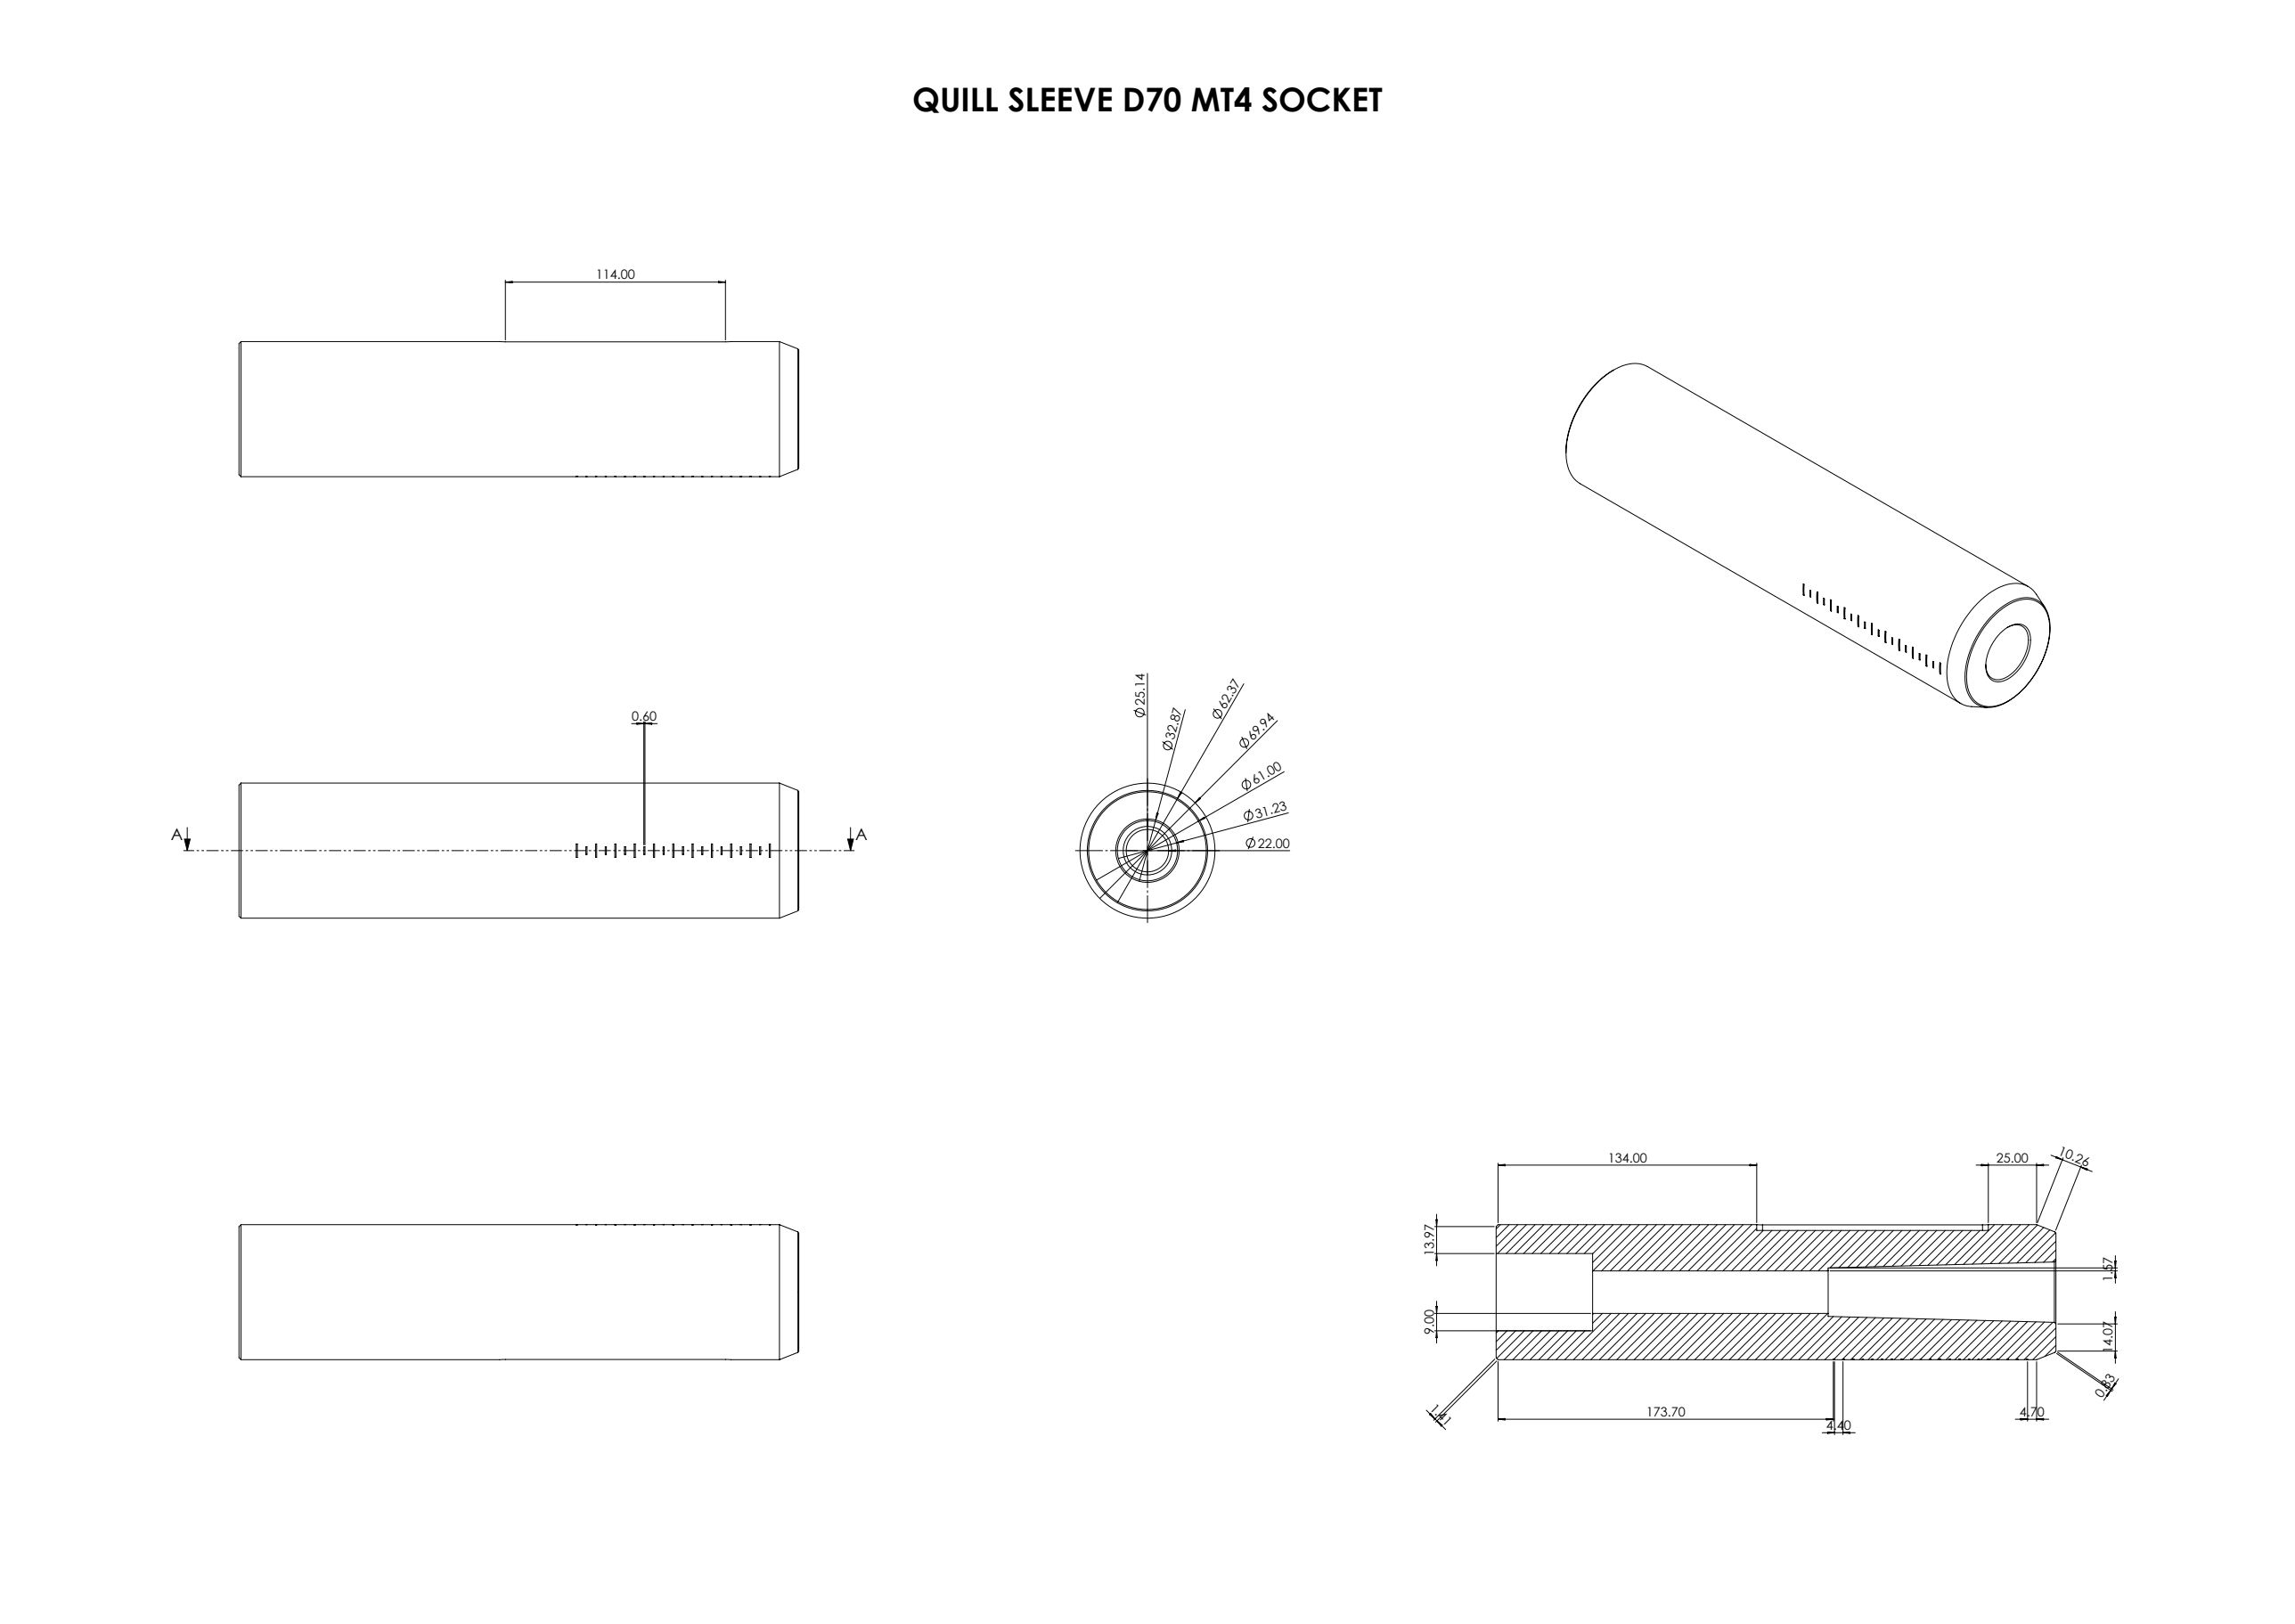
ISO-10303-21;
HEADER;
/* Generated by software containing ST-Developer
 * from STEP Tools, Inc. (www.steptools.com) 
 */

FILE_DESCRIPTION(
/* description */ (''),
/* implementation_level */ '2;1');

FILE_NAME(
/* name */ '03_Quill_Sleeve_D70_MT4_Socket.step',
/* time_stamp */ '2026-10-26T03:50:32-07:00',
/* author */ (''),
/* organization */ (''),
/* preprocessor_version */ 'ST-DEVELOPER v20.2',
/* originating_system */ 'Autodesk Translation Framework v15.15.0.0',
/* authorisation */ '');

FILE_SCHEMA (('AUTOMOTIVE_DESIGN { 1 0 10303 214 3 1 1 }'));
ENDSEC;

DATA;
#10=MECHANICAL_DESIGN_GEOMETRIC_PRESENTATION_REPRESENTATION('',(#1041),#76660);
#237=B_SPLINE_CURVE_WITH_KNOTS('',3,(#39988,#39989,#39990,#39991,#39992,
#39993,#39994,#39995,#39996,#39997,#39998,#39999,#40000,#40001,#40002,#40003,
#40004,#40005),.UNSPECIFIED.,.F.,.F.,(4,2,2,2,2,2,2,2,4),(0.,0.113065755992561,
0.226131511985123,0.3391970600484,0.452262608111676,0.565328156174953,0.67839370423823,
0.791459460230791,0.904525216223353),.UNSPECIFIED.);
#238=B_SPLINE_CURVE_WITH_KNOTS('',3,(#40016,#40017,#40018,#40019,#40020,
#40021,#40022,#40023,#40024,#40025,#40026,#40027,#40028,#40029,#40030,#40031,
#40032,#40033),.UNSPECIFIED.,.F.,.F.,(4,2,2,2,2,2,2,2,4),(-0.904525216223347,
-0.791459460230787,-0.678393704238228,-0.565328156174951,-0.452262608111673,
-0.339197060048396,-0.226131511985119,-0.11306575599256,0.),
 .UNSPECIFIED.);
#1001=SHAPE_REPRESENTATION_RELATIONSHIP('SRR','None',#76738,#1021);
#1021=ADVANCED_BREP_SHAPE_REPRESENTATION('',(#1061),#76642);
#1041=STYLED_ITEM('',(#76920),#1061);
#1061=MANIFOLD_SOLID_BREP('Quill',#26666);
#1155=CYLINDRICAL_SURFACE('',#27552,0.3);
#1156=CYLINDRICAL_SURFACE('',#27555,0.3);
#1157=CYLINDRICAL_SURFACE('',#27558,2.);
#1158=CYLINDRICAL_SURFACE('',#27565,3.497);
#1159=CYLINDRICAL_SURFACE('',#27572,1.1);
#1580=FACE_BOUND('',#4415,.T.);
#1581=FACE_BOUND('',#4528,.T.);
#1582=FACE_BOUND('',#4531,.T.);
#1583=FACE_BOUND('',#4532,.T.);
#1584=FACE_BOUND('',#4533,.T.);
#1585=FACE_BOUND('',#4534,.T.);
#1586=FACE_BOUND('',#4535,.T.);
#1587=FACE_BOUND('',#4536,.T.);
#1588=FACE_BOUND('',#4537,.T.);
#1589=FACE_BOUND('',#4538,.T.);
#1590=FACE_BOUND('',#4539,.T.);
#1591=FACE_BOUND('',#4540,.T.);
#1592=FACE_BOUND('',#4541,.T.);
#1593=FACE_BOUND('',#4542,.T.);
#1594=FACE_BOUND('',#4543,.T.);
#1595=FACE_BOUND('',#4544,.T.);
#1596=FACE_BOUND('',#4545,.T.);
#1597=FACE_BOUND('',#4546,.T.);
#1598=FACE_BOUND('',#4547,.T.);
#1599=FACE_BOUND('',#4548,.T.);
#1600=FACE_BOUND('',#4549,.T.);
#1601=FACE_BOUND('',#4550,.T.);
#1602=FACE_BOUND('',#4551,.T.);
#1603=FACE_BOUND('',#4552,.T.);
#1604=FACE_BOUND('',#4556,.T.);
#1605=FACE_BOUND('',#4559,.T.);
#1804=PLANE('',#27402);
#1805=PLANE('',#27404);
#1806=PLANE('',#27405);
#1807=PLANE('',#27407);
#1808=PLANE('',#27408);
#1809=PLANE('',#27410);
#1810=PLANE('',#27411);
#1811=PLANE('',#27412);
#1812=PLANE('',#27414);
#1813=PLANE('',#27415);
#1814=PLANE('',#27417);
#1815=PLANE('',#27418);
#1816=PLANE('',#27419);
#1817=PLANE('',#27421);
#1818=PLANE('',#27422);
#1819=PLANE('',#27424);
#1820=PLANE('',#27425);
#1821=PLANE('',#27426);
#1822=PLANE('',#27428);
#1823=PLANE('',#27429);
#1824=PLANE('',#27431);
#1825=PLANE('',#27432);
#1826=PLANE('',#27433);
#1827=PLANE('',#27435);
#1828=PLANE('',#27436);
#1829=PLANE('',#27438);
#1830=PLANE('',#27439);
#1831=PLANE('',#27440);
#1832=PLANE('',#27442);
#1833=PLANE('',#27443);
#1834=PLANE('',#27445);
#1835=PLANE('',#27446);
#1836=PLANE('',#27447);
#1837=PLANE('',#27449);
#1838=PLANE('',#27450);
#1839=PLANE('',#27452);
#1840=PLANE('',#27453);
#1841=PLANE('',#27454);
#1842=PLANE('',#27456);
#1843=PLANE('',#27457);
#1844=PLANE('',#27459);
#1845=PLANE('',#27460);
#1846=PLANE('',#27461);
#1847=PLANE('',#27463);
#1848=PLANE('',#27464);
#1849=PLANE('',#27466);
#1850=PLANE('',#27467);
#1851=PLANE('',#27468);
#1852=PLANE('',#27470);
#1853=PLANE('',#27471);
#1854=PLANE('',#27473);
#1855=PLANE('',#27474);
#1856=PLANE('',#27475);
#1857=PLANE('',#27477);
#1858=PLANE('',#27478);
#1859=PLANE('',#27480);
#1860=PLANE('',#27481);
#1861=PLANE('',#27482);
#1862=PLANE('',#27484);
#1863=PLANE('',#27485);
#1864=PLANE('',#27487);
#1865=PLANE('',#27488);
#1866=PLANE('',#27489);
#1867=PLANE('',#27491);
#1868=PLANE('',#27492);
#1869=PLANE('',#27494);
#1870=PLANE('',#27495);
#1871=PLANE('',#27496);
#1872=PLANE('',#27498);
#1873=PLANE('',#27499);
#1874=PLANE('',#27501);
#1875=PLANE('',#27502);
#1876=PLANE('',#27503);
#1877=PLANE('',#27505);
#1878=PLANE('',#27506);
#1879=PLANE('',#27508);
#1880=PLANE('',#27509);
#1881=PLANE('',#27510);
#1882=PLANE('',#27512);
#1883=PLANE('',#27513);
#1884=PLANE('',#27515);
#1885=PLANE('',#27516);
#1886=PLANE('',#27517);
#1887=PLANE('',#27519);
#1888=PLANE('',#27520);
#1889=PLANE('',#27522);
#1890=PLANE('',#27523);
#1891=PLANE('',#27524);
#1892=PLANE('',#27526);
#1893=PLANE('',#27527);
#1894=PLANE('',#27529);
#1895=PLANE('',#27530);
#1896=PLANE('',#27531);
#1897=PLANE('',#27533);
#1898=PLANE('',#27534);
#1899=PLANE('',#27536);
#1900=PLANE('',#27537);
#1901=PLANE('',#27538);
#1902=PLANE('',#27540);
#1903=PLANE('',#27541);
#1904=PLANE('',#27543);
#1905=PLANE('',#27544);
#1906=PLANE('',#27545);
#1907=PLANE('',#27547);
#1908=PLANE('',#27548);
#1909=PLANE('',#27550);
#1910=PLANE('',#27551);
#1911=PLANE('',#27554);
#1912=PLANE('',#27557);
#1913=PLANE('',#27561);
#1914=PLANE('',#27570);
#1915=PLANE('',#27574);
#2833=FACE_OUTER_BOUND('',#4412,.T.);
#2834=FACE_OUTER_BOUND('',#4413,.T.);
#2835=FACE_OUTER_BOUND('',#4414,.T.);
#2836=FACE_OUTER_BOUND('',#4416,.T.);
#2837=FACE_OUTER_BOUND('',#4417,.T.);
#2838=FACE_OUTER_BOUND('',#4418,.T.);
#2839=FACE_OUTER_BOUND('',#4419,.T.);
#2840=FACE_OUTER_BOUND('',#4420,.T.);
#2841=FACE_OUTER_BOUND('',#4421,.T.);
#2842=FACE_OUTER_BOUND('',#4422,.T.);
#2843=FACE_OUTER_BOUND('',#4423,.T.);
#2844=FACE_OUTER_BOUND('',#4424,.T.);
#2845=FACE_OUTER_BOUND('',#4425,.T.);
#2846=FACE_OUTER_BOUND('',#4426,.T.);
#2847=FACE_OUTER_BOUND('',#4427,.T.);
#2848=FACE_OUTER_BOUND('',#4428,.T.);
#2849=FACE_OUTER_BOUND('',#4429,.T.);
#2850=FACE_OUTER_BOUND('',#4430,.T.);
#2851=FACE_OUTER_BOUND('',#4431,.T.);
#2852=FACE_OUTER_BOUND('',#4432,.T.);
#2853=FACE_OUTER_BOUND('',#4433,.T.);
#2854=FACE_OUTER_BOUND('',#4434,.T.);
#2855=FACE_OUTER_BOUND('',#4435,.T.);
#2856=FACE_OUTER_BOUND('',#4436,.T.);
#2857=FACE_OUTER_BOUND('',#4437,.T.);
#2858=FACE_OUTER_BOUND('',#4438,.T.);
#2859=FACE_OUTER_BOUND('',#4439,.T.);
#2860=FACE_OUTER_BOUND('',#4440,.T.);
#2861=FACE_OUTER_BOUND('',#4441,.T.);
#2862=FACE_OUTER_BOUND('',#4442,.T.);
#2863=FACE_OUTER_BOUND('',#4443,.T.);
#2864=FACE_OUTER_BOUND('',#4444,.T.);
#2865=FACE_OUTER_BOUND('',#4445,.T.);
#2866=FACE_OUTER_BOUND('',#4446,.T.);
#2867=FACE_OUTER_BOUND('',#4447,.T.);
#2868=FACE_OUTER_BOUND('',#4448,.T.);
#2869=FACE_OUTER_BOUND('',#4449,.T.);
#2870=FACE_OUTER_BOUND('',#4450,.T.);
#2871=FACE_OUTER_BOUND('',#4451,.T.);
#2872=FACE_OUTER_BOUND('',#4452,.T.);
#2873=FACE_OUTER_BOUND('',#4453,.T.);
#2874=FACE_OUTER_BOUND('',#4454,.T.);
#2875=FACE_OUTER_BOUND('',#4455,.T.);
#2876=FACE_OUTER_BOUND('',#4456,.T.);
#2877=FACE_OUTER_BOUND('',#4457,.T.);
#2878=FACE_OUTER_BOUND('',#4458,.T.);
#2879=FACE_OUTER_BOUND('',#4459,.T.);
#2880=FACE_OUTER_BOUND('',#4460,.T.);
#2881=FACE_OUTER_BOUND('',#4461,.T.);
#2882=FACE_OUTER_BOUND('',#4462,.T.);
#2883=FACE_OUTER_BOUND('',#4463,.T.);
#2884=FACE_OUTER_BOUND('',#4464,.T.);
#2885=FACE_OUTER_BOUND('',#4465,.T.);
#2886=FACE_OUTER_BOUND('',#4466,.T.);
#2887=FACE_OUTER_BOUND('',#4467,.T.);
#2888=FACE_OUTER_BOUND('',#4468,.T.);
#2889=FACE_OUTER_BOUND('',#4469,.T.);
#2890=FACE_OUTER_BOUND('',#4470,.T.);
#2891=FACE_OUTER_BOUND('',#4471,.T.);
#2892=FACE_OUTER_BOUND('',#4472,.T.);
#2893=FACE_OUTER_BOUND('',#4473,.T.);
#2894=FACE_OUTER_BOUND('',#4474,.T.);
#2895=FACE_OUTER_BOUND('',#4475,.T.);
#2896=FACE_OUTER_BOUND('',#4476,.T.);
#2897=FACE_OUTER_BOUND('',#4477,.T.);
#2898=FACE_OUTER_BOUND('',#4478,.T.);
#2899=FACE_OUTER_BOUND('',#4479,.T.);
#2900=FACE_OUTER_BOUND('',#4480,.T.);
#2901=FACE_OUTER_BOUND('',#4481,.T.);
#2902=FACE_OUTER_BOUND('',#4482,.T.);
#2903=FACE_OUTER_BOUND('',#4483,.T.);
#2904=FACE_OUTER_BOUND('',#4484,.T.);
#2905=FACE_OUTER_BOUND('',#4485,.T.);
#2906=FACE_OUTER_BOUND('',#4486,.T.);
#2907=FACE_OUTER_BOUND('',#4487,.T.);
#2908=FACE_OUTER_BOUND('',#4488,.T.);
#2909=FACE_OUTER_BOUND('',#4489,.T.);
#2910=FACE_OUTER_BOUND('',#4490,.T.);
#2911=FACE_OUTER_BOUND('',#4491,.T.);
#2912=FACE_OUTER_BOUND('',#4492,.T.);
#2913=FACE_OUTER_BOUND('',#4493,.T.);
#2914=FACE_OUTER_BOUND('',#4494,.T.);
#2915=FACE_OUTER_BOUND('',#4495,.T.);
#2916=FACE_OUTER_BOUND('',#4496,.T.);
#2917=FACE_OUTER_BOUND('',#4497,.T.);
#2918=FACE_OUTER_BOUND('',#4498,.T.);
#2919=FACE_OUTER_BOUND('',#4499,.T.);
#2920=FACE_OUTER_BOUND('',#4500,.T.);
#2921=FACE_OUTER_BOUND('',#4501,.T.);
#2922=FACE_OUTER_BOUND('',#4502,.T.);
#2923=FACE_OUTER_BOUND('',#4503,.T.);
#2924=FACE_OUTER_BOUND('',#4504,.T.);
#2925=FACE_OUTER_BOUND('',#4505,.T.);
#2926=FACE_OUTER_BOUND('',#4506,.T.);
#2927=FACE_OUTER_BOUND('',#4507,.T.);
#2928=FACE_OUTER_BOUND('',#4508,.T.);
#2929=FACE_OUTER_BOUND('',#4509,.T.);
#2930=FACE_OUTER_BOUND('',#4510,.T.);
#2931=FACE_OUTER_BOUND('',#4511,.T.);
#2932=FACE_OUTER_BOUND('',#4512,.T.);
#2933=FACE_OUTER_BOUND('',#4513,.T.);
#2934=FACE_OUTER_BOUND('',#4514,.T.);
#2935=FACE_OUTER_BOUND('',#4515,.T.);
#2936=FACE_OUTER_BOUND('',#4516,.T.);
#2937=FACE_OUTER_BOUND('',#4517,.T.);
#2938=FACE_OUTER_BOUND('',#4518,.T.);
#2939=FACE_OUTER_BOUND('',#4519,.T.);
#2940=FACE_OUTER_BOUND('',#4520,.T.);
#2941=FACE_OUTER_BOUND('',#4521,.T.);
#2942=FACE_OUTER_BOUND('',#4522,.T.);
#2943=FACE_OUTER_BOUND('',#4523,.T.);
#2944=FACE_OUTER_BOUND('',#4524,.T.);
#2945=FACE_OUTER_BOUND('',#4525,.T.);
#2946=FACE_OUTER_BOUND('',#4526,.T.);
#2947=FACE_OUTER_BOUND('',#4527,.T.);
#2948=FACE_OUTER_BOUND('',#4529,.T.);
#2949=FACE_OUTER_BOUND('',#4530,.T.);
#2950=FACE_OUTER_BOUND('',#4553,.T.);
#2951=FACE_OUTER_BOUND('',#4554,.T.);
#2952=FACE_OUTER_BOUND('',#4555,.T.);
#2953=FACE_OUTER_BOUND('',#4557,.T.);
#2954=FACE_OUTER_BOUND('',#4558,.T.);
#4412=EDGE_LOOP('',(#18651,#18652,#18653,#18654,#18655));
#4413=EDGE_LOOP('',(#18656,#18657,#18658,#18659,#18660));
#4414=EDGE_LOOP('',(#18661));
#4415=EDGE_LOOP('',(#18662));
#4416=EDGE_LOOP('',(#18663,#18664,#18665,#18666));
#4417=EDGE_LOOP('',(#18667,#18668,#18669,#18670));
#4418=EDGE_LOOP('',(#18671,#18672,#18673,#18674));
#4419=EDGE_LOOP('',(#18675,#18676,#18677,#18678));
#4420=EDGE_LOOP('',(#18679,#18680,#18681,#18682));
#4421=EDGE_LOOP('',(#18683,#18684,#18685,#18686));
#4422=EDGE_LOOP('',(#18687,#18688,#18689,#18690));
#4423=EDGE_LOOP('',(#18691,#18692,#18693,#18694));
#4424=EDGE_LOOP('',(#18695,#18696,#18697,#18698));
#4425=EDGE_LOOP('',(#18699,#18700,#18701,#18702));
#4426=EDGE_LOOP('',(#18703,#18704,#18705,#18706));
#4427=EDGE_LOOP('',(#18707,#18708,#18709,#18710));
#4428=EDGE_LOOP('',(#18711,#18712,#18713,#18714));
#4429=EDGE_LOOP('',(#18715,#18716,#18717,#18718));
#4430=EDGE_LOOP('',(#18719,#18720,#18721,#18722));
#4431=EDGE_LOOP('',(#18723,#18724,#18725,#18726));
#4432=EDGE_LOOP('',(#18727,#18728,#18729,#18730));
#4433=EDGE_LOOP('',(#18731,#18732,#18733,#18734));
#4434=EDGE_LOOP('',(#18735,#18736,#18737,#18738));
#4435=EDGE_LOOP('',(#18739,#18740,#18741,#18742));
#4436=EDGE_LOOP('',(#18743,#18744,#18745,#18746));
#4437=EDGE_LOOP('',(#18747,#18748,#18749,#18750));
#4438=EDGE_LOOP('',(#18751,#18752,#18753,#18754));
#4439=EDGE_LOOP('',(#18755,#18756,#18757,#18758));
#4440=EDGE_LOOP('',(#18759,#18760,#18761,#18762));
#4441=EDGE_LOOP('',(#18763,#18764,#18765,#18766));
#4442=EDGE_LOOP('',(#18767,#18768,#18769,#18770));
#4443=EDGE_LOOP('',(#18771,#18772,#18773,#18774));
#4444=EDGE_LOOP('',(#18775,#18776,#18777,#18778));
#4445=EDGE_LOOP('',(#18779,#18780,#18781,#18782));
#4446=EDGE_LOOP('',(#18783,#18784,#18785,#18786));
#4447=EDGE_LOOP('',(#18787,#18788,#18789,#18790));
#4448=EDGE_LOOP('',(#18791,#18792,#18793,#18794));
#4449=EDGE_LOOP('',(#18795,#18796,#18797,#18798));
#4450=EDGE_LOOP('',(#18799,#18800,#18801,#18802));
#4451=EDGE_LOOP('',(#18803,#18804,#18805,#18806));
#4452=EDGE_LOOP('',(#18807,#18808,#18809,#18810));
#4453=EDGE_LOOP('',(#18811,#18812,#18813,#18814));
#4454=EDGE_LOOP('',(#18815,#18816,#18817,#18818));
#4455=EDGE_LOOP('',(#18819,#18820,#18821,#18822));
#4456=EDGE_LOOP('',(#18823,#18824,#18825,#18826));
#4457=EDGE_LOOP('',(#18827,#18828,#18829,#18830));
#4458=EDGE_LOOP('',(#18831,#18832,#18833,#18834));
#4459=EDGE_LOOP('',(#18835,#18836,#18837,#18838));
#4460=EDGE_LOOP('',(#18839,#18840,#18841,#18842));
#4461=EDGE_LOOP('',(#18843,#18844,#18845,#18846));
#4462=EDGE_LOOP('',(#18847,#18848,#18849,#18850));
#4463=EDGE_LOOP('',(#18851,#18852,#18853,#18854));
#4464=EDGE_LOOP('',(#18855,#18856,#18857,#18858));
#4465=EDGE_LOOP('',(#18859,#18860,#18861,#18862));
#4466=EDGE_LOOP('',(#18863,#18864,#18865,#18866));
#4467=EDGE_LOOP('',(#18867,#18868,#18869,#18870));
#4468=EDGE_LOOP('',(#18871,#18872,#18873,#18874));
#4469=EDGE_LOOP('',(#18875,#18876,#18877,#18878));
#4470=EDGE_LOOP('',(#18879,#18880,#18881,#18882));
#4471=EDGE_LOOP('',(#18883,#18884,#18885,#18886));
#4472=EDGE_LOOP('',(#18887,#18888,#18889,#18890));
#4473=EDGE_LOOP('',(#18891,#18892,#18893,#18894));
#4474=EDGE_LOOP('',(#18895,#18896,#18897,#18898));
#4475=EDGE_LOOP('',(#18899,#18900,#18901,#18902));
#4476=EDGE_LOOP('',(#18903,#18904,#18905,#18906));
#4477=EDGE_LOOP('',(#18907,#18908,#18909,#18910));
#4478=EDGE_LOOP('',(#18911,#18912,#18913,#18914));
#4479=EDGE_LOOP('',(#18915,#18916,#18917,#18918));
#4480=EDGE_LOOP('',(#18919,#18920,#18921,#18922));
#4481=EDGE_LOOP('',(#18923,#18924,#18925,#18926));
#4482=EDGE_LOOP('',(#18927,#18928,#18929,#18930));
#4483=EDGE_LOOP('',(#18931,#18932,#18933,#18934));
#4484=EDGE_LOOP('',(#18935,#18936,#18937,#18938));
#4485=EDGE_LOOP('',(#18939,#18940,#18941,#18942));
#4486=EDGE_LOOP('',(#18943,#18944,#18945,#18946));
#4487=EDGE_LOOP('',(#18947,#18948,#18949,#18950));
#4488=EDGE_LOOP('',(#18951,#18952,#18953,#18954));
#4489=EDGE_LOOP('',(#18955,#18956,#18957,#18958));
#4490=EDGE_LOOP('',(#18959,#18960,#18961,#18962));
#4491=EDGE_LOOP('',(#18963,#18964,#18965,#18966));
#4492=EDGE_LOOP('',(#18967,#18968,#18969,#18970));
#4493=EDGE_LOOP('',(#18971,#18972,#18973,#18974));
#4494=EDGE_LOOP('',(#18975,#18976,#18977,#18978));
#4495=EDGE_LOOP('',(#18979,#18980,#18981,#18982));
#4496=EDGE_LOOP('',(#18983,#18984,#18985,#18986));
#4497=EDGE_LOOP('',(#18987,#18988,#18989,#18990));
#4498=EDGE_LOOP('',(#18991,#18992,#18993,#18994));
#4499=EDGE_LOOP('',(#18995,#18996,#18997,#18998));
#4500=EDGE_LOOP('',(#18999,#19000,#19001,#19002));
#4501=EDGE_LOOP('',(#19003,#19004,#19005,#19006));
#4502=EDGE_LOOP('',(#19007,#19008,#19009,#19010));
#4503=EDGE_LOOP('',(#19011,#19012,#19013,#19014));
#4504=EDGE_LOOP('',(#19015,#19016,#19017,#19018));
#4505=EDGE_LOOP('',(#19019,#19020,#19021,#19022));
#4506=EDGE_LOOP('',(#19023,#19024,#19025,#19026));
#4507=EDGE_LOOP('',(#19027,#19028,#19029,#19030));
#4508=EDGE_LOOP('',(#19031,#19032,#19033,#19034));
#4509=EDGE_LOOP('',(#19035,#19036,#19037,#19038));
#4510=EDGE_LOOP('',(#19039,#19040,#19041,#19042));
#4511=EDGE_LOOP('',(#19043,#19044,#19045,#19046));
#4512=EDGE_LOOP('',(#19047,#19048,#19049,#19050));
#4513=EDGE_LOOP('',(#19051,#19052,#19053,#19054));
#4514=EDGE_LOOP('',(#19055,#19056,#19057,#19058));
#4515=EDGE_LOOP('',(#19059,#19060,#19061,#19062));
#4516=EDGE_LOOP('',(#19063,#19064,#19065,#19066));
#4517=EDGE_LOOP('',(#19067,#19068,#19069,#19070));
#4518=EDGE_LOOP('',(#19071,#19072,#19073,#19074));
#4519=EDGE_LOOP('',(#19075,#19076,#19077,#19078));
#4520=EDGE_LOOP('',(#19079,#19080,#19081,#19082));
#4521=EDGE_LOOP('',(#19083,#19084,#19085,#19086));
#4522=EDGE_LOOP('',(#19087,#19088,#19089,#19090));
#4523=EDGE_LOOP('',(#19091,#19092,#19093,#19094));
#4524=EDGE_LOOP('',(#19095,#19096,#19097,#19098));
#4525=EDGE_LOOP('',(#19099,#19100,#19101,#19102));
#4526=EDGE_LOOP('',(#19103,#19104,#19105,#19106));
#4527=EDGE_LOOP('',(#19107));
#4528=EDGE_LOOP('',(#19108));
#4529=EDGE_LOOP('',(#19109,#19110,#19111,#19112));
#4530=EDGE_LOOP('',(#19113,#19114,#19115,#19116));
#4531=EDGE_LOOP('',(#19117,#19118,#19119,#19120));
#4532=EDGE_LOOP('',(#19121,#19122,#19123,#19124));
#4533=EDGE_LOOP('',(#19125,#19126,#19127,#19128));
#4534=EDGE_LOOP('',(#19129,#19130,#19131,#19132));
#4535=EDGE_LOOP('',(#19133,#19134,#19135,#19136));
#4536=EDGE_LOOP('',(#19137,#19138,#19139,#19140));
#4537=EDGE_LOOP('',(#19141,#19142,#19143,#19144));
#4538=EDGE_LOOP('',(#19145,#19146,#19147,#19148));
#4539=EDGE_LOOP('',(#19149,#19150,#19151,#19152));
#4540=EDGE_LOOP('',(#19153,#19154,#19155,#19156));
#4541=EDGE_LOOP('',(#19157,#19158,#19159,#19160));
#4542=EDGE_LOOP('',(#19161,#19162,#19163,#19164));
#4543=EDGE_LOOP('',(#19165,#19166,#19167,#19168));
#4544=EDGE_LOOP('',(#19169,#19170,#19171,#19172));
#4545=EDGE_LOOP('',(#19173,#19174,#19175,#19176));
#4546=EDGE_LOOP('',(#19177,#19178,#19179,#19180));
#4547=EDGE_LOOP('',(#19181,#19182,#19183,#19184));
#4548=EDGE_LOOP('',(#19185,#19186,#19187,#19188));
#4549=EDGE_LOOP('',(#19189,#19190,#19191,#19192));
#4550=EDGE_LOOP('',(#19193,#19194,#19195,#19196));
#4551=EDGE_LOOP('',(#19197,#19198,#19199,#19200));
#4552=EDGE_LOOP('',(#19201,#19202,#19203,#19204));
#4553=EDGE_LOOP('',(#19205,#19206,#19207,#19208));
#4554=EDGE_LOOP('',(#19209,#19210,#19211,#19212));
#4555=EDGE_LOOP('',(#19213));
#4556=EDGE_LOOP('',(#19214));
#4557=EDGE_LOOP('',(#19215,#19216,#19217,#19218));
#4558=EDGE_LOOP('',(#19219));
#4559=EDGE_LOOP('',(#19220));
#5919=CIRCLE('',#27397,3.05);
#5920=CIRCLE('',#27398,3.11844928601987);
#5921=CIRCLE('',#27399,3.11844928601987);
#5922=CIRCLE('',#27401,3.497);
#5923=CIRCLE('',#27403,1.64335);
#5924=CIRCLE('',#27406,3.497);
#5925=CIRCLE('',#27409,3.497);
#5926=CIRCLE('',#27413,3.497);
#5927=CIRCLE('',#27416,3.497);
#5928=CIRCLE('',#27420,3.497);
#5929=CIRCLE('',#27423,3.497);
#5930=CIRCLE('',#27427,3.497);
#5931=CIRCLE('',#27430,3.497);
#5932=CIRCLE('',#27434,3.497);
#5933=CIRCLE('',#27437,3.497);
#5934=CIRCLE('',#27441,3.497);
#5935=CIRCLE('',#27444,3.497);
#5936=CIRCLE('',#27448,3.497);
#5937=CIRCLE('',#27451,3.497);
#5938=CIRCLE('',#27455,3.497);
#5939=CIRCLE('',#27458,3.497);
#5940=CIRCLE('',#27462,3.497);
#5941=CIRCLE('',#27465,3.497);
#5942=CIRCLE('',#27469,3.497);
#5943=CIRCLE('',#27472,3.497);
#5944=CIRCLE('',#27476,3.497);
#5945=CIRCLE('',#27479,3.497);
#5946=CIRCLE('',#27483,3.497);
#5947=CIRCLE('',#27486,3.497);
#5948=CIRCLE('',#27490,3.497);
#5949=CIRCLE('',#27493,3.497);
#5950=CIRCLE('',#27497,3.497);
#5951=CIRCLE('',#27500,3.497);
#5952=CIRCLE('',#27504,3.497);
#5953=CIRCLE('',#27507,3.497);
#5954=CIRCLE('',#27511,3.497);
#5955=CIRCLE('',#27514,3.497);
#5956=CIRCLE('',#27518,3.497);
#5957=CIRCLE('',#27521,3.497);
#5958=CIRCLE('',#27525,3.497);
#5959=CIRCLE('',#27528,3.497);
#5960=CIRCLE('',#27532,3.497);
#5961=CIRCLE('',#27535,3.497);
#5962=CIRCLE('',#27539,3.497);
#5963=CIRCLE('',#27542,3.497);
#5964=CIRCLE('',#27546,3.497);
#5965=CIRCLE('',#27549,3.497);
#5966=CIRCLE('',#27553,0.3);
#5967=CIRCLE('',#27556,0.3);
#5968=CIRCLE('',#27559,2.);
#5969=CIRCLE('',#27560,2.);
#5970=CIRCLE('',#27562,3.397);
#5971=CIRCLE('',#27564,3.497);
#5972=CIRCLE('',#27567,1.5612724);
#5973=CIRCLE('',#27569,1.256904);
#5974=CIRCLE('',#27571,1.1);
#5975=CIRCLE('',#27573,1.1);
#7064=LINE('',#39441,#9220);
#7065=LINE('',#39447,#9221);
#7066=LINE('',#39455,#9222);
#7067=LINE('',#39457,#9223);
#7068=LINE('',#39459,#9224);
#7069=LINE('',#39460,#9225);
#7070=LINE('',#39465,#9226);
#7071=LINE('',#39466,#9227);
#7072=LINE('',#39469,#9228);
#7073=LINE('',#39471,#9229);
#7074=LINE('',#39472,#9230);
#7075=LINE('',#39475,#9231);
#7076=LINE('',#39480,#9232);
#7077=LINE('',#39482,#9233);
#7078=LINE('',#39484,#9234);
#7079=LINE('',#39485,#9235);
#7080=LINE('',#39490,#9236);
#7081=LINE('',#39491,#9237);
#7082=LINE('',#39494,#9238);
#7083=LINE('',#39496,#9239);
#7084=LINE('',#39497,#9240);
#7085=LINE('',#39500,#9241);
#7086=LINE('',#39505,#9242);
#7087=LINE('',#39507,#9243);
#7088=LINE('',#39509,#9244);
#7089=LINE('',#39510,#9245);
#7090=LINE('',#39515,#9246);
#7091=LINE('',#39516,#9247);
#7092=LINE('',#39519,#9248);
#7093=LINE('',#39521,#9249);
#7094=LINE('',#39522,#9250);
#7095=LINE('',#39525,#9251);
#7096=LINE('',#39530,#9252);
#7097=LINE('',#39532,#9253);
#7098=LINE('',#39534,#9254);
#7099=LINE('',#39535,#9255);
#7100=LINE('',#39540,#9256);
#7101=LINE('',#39541,#9257);
#7102=LINE('',#39544,#9258);
#7103=LINE('',#39546,#9259);
#7104=LINE('',#39547,#9260);
#7105=LINE('',#39550,#9261);
#7106=LINE('',#39555,#9262);
#7107=LINE('',#39557,#9263);
#7108=LINE('',#39559,#9264);
#7109=LINE('',#39560,#9265);
#7110=LINE('',#39565,#9266);
#7111=LINE('',#39566,#9267);
#7112=LINE('',#39569,#9268);
#7113=LINE('',#39571,#9269);
#7114=LINE('',#39572,#9270);
#7115=LINE('',#39575,#9271);
#7116=LINE('',#39580,#9272);
#7117=LINE('',#39582,#9273);
#7118=LINE('',#39584,#9274);
#7119=LINE('',#39585,#9275);
#7120=LINE('',#39590,#9276);
#7121=LINE('',#39591,#9277);
#7122=LINE('',#39594,#9278);
#7123=LINE('',#39596,#9279);
#7124=LINE('',#39597,#9280);
#7125=LINE('',#39600,#9281);
#7126=LINE('',#39605,#9282);
#7127=LINE('',#39607,#9283);
#7128=LINE('',#39609,#9284);
#7129=LINE('',#39610,#9285);
#7130=LINE('',#39615,#9286);
#7131=LINE('',#39616,#9287);
#7132=LINE('',#39619,#9288);
#7133=LINE('',#39621,#9289);
#7134=LINE('',#39622,#9290);
#7135=LINE('',#39625,#9291);
#7136=LINE('',#39630,#9292);
#7137=LINE('',#39632,#9293);
#7138=LINE('',#39634,#9294);
#7139=LINE('',#39635,#9295);
#7140=LINE('',#39640,#9296);
#7141=LINE('',#39641,#9297);
#7142=LINE('',#39644,#9298);
#7143=LINE('',#39646,#9299);
#7144=LINE('',#39647,#9300);
#7145=LINE('',#39650,#9301);
#7146=LINE('',#39655,#9302);
#7147=LINE('',#39657,#9303);
#7148=LINE('',#39659,#9304);
#7149=LINE('',#39660,#9305);
#7150=LINE('',#39665,#9306);
#7151=LINE('',#39666,#9307);
#7152=LINE('',#39669,#9308);
#7153=LINE('',#39671,#9309);
#7154=LINE('',#39672,#9310);
#7155=LINE('',#39675,#9311);
#7156=LINE('',#39680,#9312);
#7157=LINE('',#39682,#9313);
#7158=LINE('',#39684,#9314);
#7159=LINE('',#39685,#9315);
#7160=LINE('',#39690,#9316);
#7161=LINE('',#39691,#9317);
#7162=LINE('',#39694,#9318);
#7163=LINE('',#39696,#9319);
#7164=LINE('',#39697,#9320);
#7165=LINE('',#39700,#9321);
#7166=LINE('',#39705,#9322);
#7167=LINE('',#39707,#9323);
#7168=LINE('',#39709,#9324);
#7169=LINE('',#39710,#9325);
#7170=LINE('',#39715,#9326);
#7171=LINE('',#39716,#9327);
#7172=LINE('',#39719,#9328);
#7173=LINE('',#39721,#9329);
#7174=LINE('',#39722,#9330);
#7175=LINE('',#39725,#9331);
#7176=LINE('',#39730,#9332);
#7177=LINE('',#39732,#9333);
#7178=LINE('',#39734,#9334);
#7179=LINE('',#39735,#9335);
#7180=LINE('',#39740,#9336);
#7181=LINE('',#39741,#9337);
#7182=LINE('',#39744,#9338);
#7183=LINE('',#39746,#9339);
#7184=LINE('',#39747,#9340);
#7185=LINE('',#39750,#9341);
#7186=LINE('',#39755,#9342);
#7187=LINE('',#39757,#9343);
#7188=LINE('',#39759,#9344);
#7189=LINE('',#39760,#9345);
#7190=LINE('',#39765,#9346);
#7191=LINE('',#39766,#9347);
#7192=LINE('',#39769,#9348);
#7193=LINE('',#39771,#9349);
#7194=LINE('',#39772,#9350);
#7195=LINE('',#39775,#9351);
#7196=LINE('',#39780,#9352);
#7197=LINE('',#39782,#9353);
#7198=LINE('',#39784,#9354);
#7199=LINE('',#39785,#9355);
#7200=LINE('',#39790,#9356);
#7201=LINE('',#39791,#9357);
#7202=LINE('',#39794,#9358);
#7203=LINE('',#39796,#9359);
#7204=LINE('',#39797,#9360);
#7205=LINE('',#39800,#9361);
#7206=LINE('',#39805,#9362);
#7207=LINE('',#39807,#9363);
#7208=LINE('',#39809,#9364);
#7209=LINE('',#39810,#9365);
#7210=LINE('',#39815,#9366);
#7211=LINE('',#39816,#9367);
#7212=LINE('',#39819,#9368);
#7213=LINE('',#39821,#9369);
#7214=LINE('',#39822,#9370);
#7215=LINE('',#39825,#9371);
#7216=LINE('',#39830,#9372);
#7217=LINE('',#39832,#9373);
#7218=LINE('',#39834,#9374);
#7219=LINE('',#39835,#9375);
#7220=LINE('',#39840,#9376);
#7221=LINE('',#39841,#9377);
#7222=LINE('',#39844,#9378);
#7223=LINE('',#39846,#9379);
#7224=LINE('',#39847,#9380);
#7225=LINE('',#39850,#9381);
#7226=LINE('',#39855,#9382);
#7227=LINE('',#39857,#9383);
#7228=LINE('',#39859,#9384);
#7229=LINE('',#39860,#9385);
#7230=LINE('',#39865,#9386);
#7231=LINE('',#39866,#9387);
#7232=LINE('',#39869,#9388);
#7233=LINE('',#39871,#9389);
#7234=LINE('',#39872,#9390);
#7235=LINE('',#39875,#9391);
#7236=LINE('',#39880,#9392);
#7237=LINE('',#39882,#9393);
#7238=LINE('',#39884,#9394);
#7239=LINE('',#39885,#9395);
#7240=LINE('',#39890,#9396);
#7241=LINE('',#39891,#9397);
#7242=LINE('',#39894,#9398);
#7243=LINE('',#39896,#9399);
#7244=LINE('',#39897,#9400);
#7245=LINE('',#39900,#9401);
#7246=LINE('',#39905,#9402);
#7247=LINE('',#39907,#9403);
#7248=LINE('',#39909,#9404);
#7249=LINE('',#39910,#9405);
#7250=LINE('',#39915,#9406);
#7251=LINE('',#39916,#9407);
#7252=LINE('',#39919,#9408);
#7253=LINE('',#39921,#9409);
#7254=LINE('',#39922,#9410);
#7255=LINE('',#39925,#9411);
#7256=LINE('',#39930,#9412);
#7257=LINE('',#39932,#9413);
#7258=LINE('',#39934,#9414);
#7259=LINE('',#39935,#9415);
#7260=LINE('',#39940,#9416);
#7261=LINE('',#39941,#9417);
#7262=LINE('',#39944,#9418);
#7263=LINE('',#39946,#9419);
#7264=LINE('',#39947,#9420);
#7265=LINE('',#39950,#9421);
#7266=LINE('',#39955,#9422);
#7267=LINE('',#39957,#9423);
#7268=LINE('',#39959,#9424);
#7269=LINE('',#39960,#9425);
#7270=LINE('',#39965,#9426);
#7271=LINE('',#39966,#9427);
#7272=LINE('',#39969,#9428);
#7273=LINE('',#39971,#9429);
#7274=LINE('',#39972,#9430);
#7275=LINE('',#39975,#9431);
#7276=LINE('',#39980,#9432);
#7277=LINE('',#39982,#9433);
#7278=LINE('',#39984,#9434);
#7279=LINE('',#39985,#9435);
#7280=LINE('',#40008,#9436);
#7281=LINE('',#40011,#9437);
#7282=LINE('',#40013,#9438);
#7283=LINE('',#40014,#9439);
#7284=LINE('',#40040,#9440);
#7285=LINE('',#40048,#9441);
#7286=LINE('',#40050,#9442);
#7287=LINE('',#40053,#9443);
#7288=LINE('',#40057,#9444);
#7289=LINE('',#40064,#9445);
#9220=VECTOR('',#30803,3.08422464300993);
#9221=VECTOR('',#30810,3.2985);
#9222=VECTOR('',#30819,1.);
#9223=VECTOR('',#30820,1.);
#9224=VECTOR('',#30821,1.);
#9225=VECTOR('',#30822,1.);
#9226=VECTOR('',#30827,1.);
#9227=VECTOR('',#30828,1.);
#9228=VECTOR('',#30831,1.);
#9229=VECTOR('',#30832,1.);
#9230=VECTOR('',#30833,1.);
#9231=VECTOR('',#30838,1.);
#9232=VECTOR('',#30843,1.);
#9233=VECTOR('',#30844,1.);
#9234=VECTOR('',#30845,1.);
#9235=VECTOR('',#30846,1.);
#9236=VECTOR('',#30851,1.);
#9237=VECTOR('',#30852,1.);
#9238=VECTOR('',#30855,1.);
#9239=VECTOR('',#30856,1.);
#9240=VECTOR('',#30857,1.);
#9241=VECTOR('',#30862,1.);
#9242=VECTOR('',#30867,1.);
#9243=VECTOR('',#30868,1.);
#9244=VECTOR('',#30869,1.);
#9245=VECTOR('',#30870,1.);
#9246=VECTOR('',#30875,1.);
#9247=VECTOR('',#30876,1.);
#9248=VECTOR('',#30879,1.);
#9249=VECTOR('',#30880,1.);
#9250=VECTOR('',#30881,1.);
#9251=VECTOR('',#30886,1.);
#9252=VECTOR('',#30891,1.);
#9253=VECTOR('',#30892,1.);
#9254=VECTOR('',#30893,1.);
#9255=VECTOR('',#30894,1.);
#9256=VECTOR('',#30899,1.);
#9257=VECTOR('',#30900,1.);
#9258=VECTOR('',#30903,1.);
#9259=VECTOR('',#30904,1.);
#9260=VECTOR('',#30905,1.);
#9261=VECTOR('',#30910,1.);
#9262=VECTOR('',#30915,1.);
#9263=VECTOR('',#30916,1.);
#9264=VECTOR('',#30917,1.);
#9265=VECTOR('',#30918,1.);
#9266=VECTOR('',#30923,1.);
#9267=VECTOR('',#30924,1.);
#9268=VECTOR('',#30927,1.);
#9269=VECTOR('',#30928,1.);
#9270=VECTOR('',#30929,1.);
#9271=VECTOR('',#30934,1.);
#9272=VECTOR('',#30939,1.);
#9273=VECTOR('',#30940,1.);
#9274=VECTOR('',#30941,1.);
#9275=VECTOR('',#30942,1.);
#9276=VECTOR('',#30947,1.);
#9277=VECTOR('',#30948,1.);
#9278=VECTOR('',#30951,1.);
#9279=VECTOR('',#30952,1.);
#9280=VECTOR('',#30953,1.);
#9281=VECTOR('',#30958,1.);
#9282=VECTOR('',#30963,1.);
#9283=VECTOR('',#30964,1.);
#9284=VECTOR('',#30965,1.);
#9285=VECTOR('',#30966,1.);
#9286=VECTOR('',#30971,1.);
#9287=VECTOR('',#30972,1.);
#9288=VECTOR('',#30975,1.);
#9289=VECTOR('',#30976,1.);
#9290=VECTOR('',#30977,1.);
#9291=VECTOR('',#30982,1.);
#9292=VECTOR('',#30987,1.);
#9293=VECTOR('',#30988,1.);
#9294=VECTOR('',#30989,1.);
#9295=VECTOR('',#30990,1.);
#9296=VECTOR('',#30995,1.);
#9297=VECTOR('',#30996,1.);
#9298=VECTOR('',#30999,1.);
#9299=VECTOR('',#31000,1.);
#9300=VECTOR('',#31001,1.);
#9301=VECTOR('',#31006,1.);
#9302=VECTOR('',#31011,1.);
#9303=VECTOR('',#31012,1.);
#9304=VECTOR('',#31013,1.);
#9305=VECTOR('',#31014,1.);
#9306=VECTOR('',#31019,1.);
#9307=VECTOR('',#31020,1.);
#9308=VECTOR('',#31023,1.);
#9309=VECTOR('',#31024,1.);
#9310=VECTOR('',#31025,1.);
#9311=VECTOR('',#31030,1.);
#9312=VECTOR('',#31035,1.);
#9313=VECTOR('',#31036,1.);
#9314=VECTOR('',#31037,1.);
#9315=VECTOR('',#31038,1.);
#9316=VECTOR('',#31043,1.);
#9317=VECTOR('',#31044,1.);
#9318=VECTOR('',#31047,1.);
#9319=VECTOR('',#31048,1.);
#9320=VECTOR('',#31049,1.);
#9321=VECTOR('',#31054,1.);
#9322=VECTOR('',#31059,1.);
#9323=VECTOR('',#31060,1.);
#9324=VECTOR('',#31061,1.);
#9325=VECTOR('',#31062,1.);
#9326=VECTOR('',#31067,1.);
#9327=VECTOR('',#31068,1.);
#9328=VECTOR('',#31071,1.);
#9329=VECTOR('',#31072,1.);
#9330=VECTOR('',#31073,1.);
#9331=VECTOR('',#31078,1.);
#9332=VECTOR('',#31083,1.);
#9333=VECTOR('',#31084,1.);
#9334=VECTOR('',#31085,1.);
#9335=VECTOR('',#31086,1.);
#9336=VECTOR('',#31091,1.);
#9337=VECTOR('',#31092,1.);
#9338=VECTOR('',#31095,1.);
#9339=VECTOR('',#31096,1.);
#9340=VECTOR('',#31097,1.);
#9341=VECTOR('',#31102,1.);
#9342=VECTOR('',#31107,1.);
#9343=VECTOR('',#31108,1.);
#9344=VECTOR('',#31109,1.);
#9345=VECTOR('',#31110,1.);
#9346=VECTOR('',#31115,1.);
#9347=VECTOR('',#31116,1.);
#9348=VECTOR('',#31119,1.);
#9349=VECTOR('',#31120,1.);
#9350=VECTOR('',#31121,1.);
#9351=VECTOR('',#31126,1.);
#9352=VECTOR('',#31131,1.);
#9353=VECTOR('',#31132,1.);
#9354=VECTOR('',#31133,1.);
#9355=VECTOR('',#31134,1.);
#9356=VECTOR('',#31139,1.);
#9357=VECTOR('',#31140,1.);
#9358=VECTOR('',#31143,1.);
#9359=VECTOR('',#31144,1.);
#9360=VECTOR('',#31145,1.);
#9361=VECTOR('',#31150,1.);
#9362=VECTOR('',#31155,1.);
#9363=VECTOR('',#31156,1.);
#9364=VECTOR('',#31157,1.);
#9365=VECTOR('',#31158,1.);
#9366=VECTOR('',#31163,1.);
#9367=VECTOR('',#31164,1.);
#9368=VECTOR('',#31167,1.);
#9369=VECTOR('',#31168,1.);
#9370=VECTOR('',#31169,1.);
#9371=VECTOR('',#31174,1.);
#9372=VECTOR('',#31179,1.);
#9373=VECTOR('',#31180,1.);
#9374=VECTOR('',#31181,1.);
#9375=VECTOR('',#31182,1.);
#9376=VECTOR('',#31187,1.);
#9377=VECTOR('',#31188,1.);
#9378=VECTOR('',#31191,1.);
#9379=VECTOR('',#31192,1.);
#9380=VECTOR('',#31193,1.);
#9381=VECTOR('',#31198,1.);
#9382=VECTOR('',#31203,1.);
#9383=VECTOR('',#31204,1.);
#9384=VECTOR('',#31205,1.);
#9385=VECTOR('',#31206,1.);
#9386=VECTOR('',#31211,1.);
#9387=VECTOR('',#31212,1.);
#9388=VECTOR('',#31215,1.);
#9389=VECTOR('',#31216,1.);
#9390=VECTOR('',#31217,1.);
#9391=VECTOR('',#31222,1.);
#9392=VECTOR('',#31227,1.);
#9393=VECTOR('',#31228,1.);
#9394=VECTOR('',#31229,1.);
#9395=VECTOR('',#31230,1.);
#9396=VECTOR('',#31235,1.);
#9397=VECTOR('',#31236,1.);
#9398=VECTOR('',#31239,1.);
#9399=VECTOR('',#31240,1.);
#9400=VECTOR('',#31241,1.);
#9401=VECTOR('',#31246,1.);
#9402=VECTOR('',#31251,1.);
#9403=VECTOR('',#31252,1.);
#9404=VECTOR('',#31253,1.);
#9405=VECTOR('',#31254,1.);
#9406=VECTOR('',#31259,1.);
#9407=VECTOR('',#31260,1.);
#9408=VECTOR('',#31263,1.);
#9409=VECTOR('',#31264,1.);
#9410=VECTOR('',#31265,1.);
#9411=VECTOR('',#31270,1.);
#9412=VECTOR('',#31275,1.);
#9413=VECTOR('',#31276,1.);
#9414=VECTOR('',#31277,1.);
#9415=VECTOR('',#31278,1.);
#9416=VECTOR('',#31283,1.);
#9417=VECTOR('',#31284,1.);
#9418=VECTOR('',#31287,1.);
#9419=VECTOR('',#31288,1.);
#9420=VECTOR('',#31289,1.);
#9421=VECTOR('',#31294,1.);
#9422=VECTOR('',#31299,1.);
#9423=VECTOR('',#31300,1.);
#9424=VECTOR('',#31301,1.);
#9425=VECTOR('',#31302,1.);
#9426=VECTOR('',#31307,1.);
#9427=VECTOR('',#31308,1.);
#9428=VECTOR('',#31311,1.);
#9429=VECTOR('',#31312,1.);
#9430=VECTOR('',#31313,1.);
#9431=VECTOR('',#31318,1.);
#9432=VECTOR('',#31323,1.);
#9433=VECTOR('',#31324,1.);
#9434=VECTOR('',#31325,1.);
#9435=VECTOR('',#31326,1.);
#9436=VECTOR('',#31331,1.);
#9437=VECTOR('',#31334,1.);
#9438=VECTOR('',#31335,1.);
#9439=VECTOR('',#31336,1.);
#9440=VECTOR('',#31347,2.);
#9441=VECTOR('',#31358,3.447);
#9442=VECTOR('',#31361,3.497);
#9443=VECTOR('',#31364,1.6023112);
#9444=VECTOR('',#31369,1.4090882);
#9445=VECTOR('',#31378,1.1);
#11337=VERTEX_POINT('',#39438);
#11338=VERTEX_POINT('',#39440);
#11339=VERTEX_POINT('',#39442);
#11340=VERTEX_POINT('',#39446);
#11341=VERTEX_POINT('',#39450);
#11342=VERTEX_POINT('',#39453);
#11343=VERTEX_POINT('',#39454);
#11344=VERTEX_POINT('',#39456);
#11345=VERTEX_POINT('',#39458);
#11346=VERTEX_POINT('',#39462);
#11347=VERTEX_POINT('',#39464);
#11348=VERTEX_POINT('',#39468);
#11349=VERTEX_POINT('',#39470);
#11350=VERTEX_POINT('',#39478);
#11351=VERTEX_POINT('',#39479);
#11352=VERTEX_POINT('',#39481);
#11353=VERTEX_POINT('',#39483);
#11354=VERTEX_POINT('',#39487);
#11355=VERTEX_POINT('',#39489);
#11356=VERTEX_POINT('',#39493);
#11357=VERTEX_POINT('',#39495);
#11358=VERTEX_POINT('',#39503);
#11359=VERTEX_POINT('',#39504);
#11360=VERTEX_POINT('',#39506);
#11361=VERTEX_POINT('',#39508);
#11362=VERTEX_POINT('',#39512);
#11363=VERTEX_POINT('',#39514);
#11364=VERTEX_POINT('',#39518);
#11365=VERTEX_POINT('',#39520);
#11366=VERTEX_POINT('',#39528);
#11367=VERTEX_POINT('',#39529);
#11368=VERTEX_POINT('',#39531);
#11369=VERTEX_POINT('',#39533);
#11370=VERTEX_POINT('',#39537);
#11371=VERTEX_POINT('',#39539);
#11372=VERTEX_POINT('',#39543);
#11373=VERTEX_POINT('',#39545);
#11374=VERTEX_POINT('',#39553);
#11375=VERTEX_POINT('',#39554);
#11376=VERTEX_POINT('',#39556);
#11377=VERTEX_POINT('',#39558);
#11378=VERTEX_POINT('',#39562);
#11379=VERTEX_POINT('',#39564);
#11380=VERTEX_POINT('',#39568);
#11381=VERTEX_POINT('',#39570);
#11382=VERTEX_POINT('',#39578);
#11383=VERTEX_POINT('',#39579);
#11384=VERTEX_POINT('',#39581);
#11385=VERTEX_POINT('',#39583);
#11386=VERTEX_POINT('',#39587);
#11387=VERTEX_POINT('',#39589);
#11388=VERTEX_POINT('',#39593);
#11389=VERTEX_POINT('',#39595);
#11390=VERTEX_POINT('',#39603);
#11391=VERTEX_POINT('',#39604);
#11392=VERTEX_POINT('',#39606);
#11393=VERTEX_POINT('',#39608);
#11394=VERTEX_POINT('',#39612);
#11395=VERTEX_POINT('',#39614);
#11396=VERTEX_POINT('',#39618);
#11397=VERTEX_POINT('',#39620);
#11398=VERTEX_POINT('',#39628);
#11399=VERTEX_POINT('',#39629);
#11400=VERTEX_POINT('',#39631);
#11401=VERTEX_POINT('',#39633);
#11402=VERTEX_POINT('',#39637);
#11403=VERTEX_POINT('',#39639);
#11404=VERTEX_POINT('',#39643);
#11405=VERTEX_POINT('',#39645);
#11406=VERTEX_POINT('',#39653);
#11407=VERTEX_POINT('',#39654);
#11408=VERTEX_POINT('',#39656);
#11409=VERTEX_POINT('',#39658);
#11410=VERTEX_POINT('',#39662);
#11411=VERTEX_POINT('',#39664);
#11412=VERTEX_POINT('',#39668);
#11413=VERTEX_POINT('',#39670);
#11414=VERTEX_POINT('',#39678);
#11415=VERTEX_POINT('',#39679);
#11416=VERTEX_POINT('',#39681);
#11417=VERTEX_POINT('',#39683);
#11418=VERTEX_POINT('',#39687);
#11419=VERTEX_POINT('',#39689);
#11420=VERTEX_POINT('',#39693);
#11421=VERTEX_POINT('',#39695);
#11422=VERTEX_POINT('',#39703);
#11423=VERTEX_POINT('',#39704);
#11424=VERTEX_POINT('',#39706);
#11425=VERTEX_POINT('',#39708);
#11426=VERTEX_POINT('',#39712);
#11427=VERTEX_POINT('',#39714);
#11428=VERTEX_POINT('',#39718);
#11429=VERTEX_POINT('',#39720);
#11430=VERTEX_POINT('',#39728);
#11431=VERTEX_POINT('',#39729);
#11432=VERTEX_POINT('',#39731);
#11433=VERTEX_POINT('',#39733);
#11434=VERTEX_POINT('',#39737);
#11435=VERTEX_POINT('',#39739);
#11436=VERTEX_POINT('',#39743);
#11437=VERTEX_POINT('',#39745);
#11438=VERTEX_POINT('',#39753);
#11439=VERTEX_POINT('',#39754);
#11440=VERTEX_POINT('',#39756);
#11441=VERTEX_POINT('',#39758);
#11442=VERTEX_POINT('',#39762);
#11443=VERTEX_POINT('',#39764);
#11444=VERTEX_POINT('',#39768);
#11445=VERTEX_POINT('',#39770);
#11446=VERTEX_POINT('',#39778);
#11447=VERTEX_POINT('',#39779);
#11448=VERTEX_POINT('',#39781);
#11449=VERTEX_POINT('',#39783);
#11450=VERTEX_POINT('',#39787);
#11451=VERTEX_POINT('',#39789);
#11452=VERTEX_POINT('',#39793);
#11453=VERTEX_POINT('',#39795);
#11454=VERTEX_POINT('',#39803);
#11455=VERTEX_POINT('',#39804);
#11456=VERTEX_POINT('',#39806);
#11457=VERTEX_POINT('',#39808);
#11458=VERTEX_POINT('',#39812);
#11459=VERTEX_POINT('',#39814);
#11460=VERTEX_POINT('',#39818);
#11461=VERTEX_POINT('',#39820);
#11462=VERTEX_POINT('',#39828);
#11463=VERTEX_POINT('',#39829);
#11464=VERTEX_POINT('',#39831);
#11465=VERTEX_POINT('',#39833);
#11466=VERTEX_POINT('',#39837);
#11467=VERTEX_POINT('',#39839);
#11468=VERTEX_POINT('',#39843);
#11469=VERTEX_POINT('',#39845);
#11470=VERTEX_POINT('',#39853);
#11471=VERTEX_POINT('',#39854);
#11472=VERTEX_POINT('',#39856);
#11473=VERTEX_POINT('',#39858);
#11474=VERTEX_POINT('',#39862);
#11475=VERTEX_POINT('',#39864);
#11476=VERTEX_POINT('',#39868);
#11477=VERTEX_POINT('',#39870);
#11478=VERTEX_POINT('',#39878);
#11479=VERTEX_POINT('',#39879);
#11480=VERTEX_POINT('',#39881);
#11481=VERTEX_POINT('',#39883);
#11482=VERTEX_POINT('',#39887);
#11483=VERTEX_POINT('',#39889);
#11484=VERTEX_POINT('',#39893);
#11485=VERTEX_POINT('',#39895);
#11486=VERTEX_POINT('',#39903);
#11487=VERTEX_POINT('',#39904);
#11488=VERTEX_POINT('',#39906);
#11489=VERTEX_POINT('',#39908);
#11490=VERTEX_POINT('',#39912);
#11491=VERTEX_POINT('',#39914);
#11492=VERTEX_POINT('',#39918);
#11493=VERTEX_POINT('',#39920);
#11494=VERTEX_POINT('',#39928);
#11495=VERTEX_POINT('',#39929);
#11496=VERTEX_POINT('',#39931);
#11497=VERTEX_POINT('',#39933);
#11498=VERTEX_POINT('',#39937);
#11499=VERTEX_POINT('',#39939);
#11500=VERTEX_POINT('',#39943);
#11501=VERTEX_POINT('',#39945);
#11502=VERTEX_POINT('',#39953);
#11503=VERTEX_POINT('',#39954);
#11504=VERTEX_POINT('',#39956);
#11505=VERTEX_POINT('',#39958);
#11506=VERTEX_POINT('',#39962);
#11507=VERTEX_POINT('',#39964);
#11508=VERTEX_POINT('',#39968);
#11509=VERTEX_POINT('',#39970);
#11510=VERTEX_POINT('',#39978);
#11511=VERTEX_POINT('',#39979);
#11512=VERTEX_POINT('',#39981);
#11513=VERTEX_POINT('',#39983);
#11514=VERTEX_POINT('',#39987);
#11515=VERTEX_POINT('',#40006);
#11516=VERTEX_POINT('',#40010);
#11517=VERTEX_POINT('',#40012);
#11518=VERTEX_POINT('',#40037);
#11519=VERTEX_POINT('',#40039);
#11520=VERTEX_POINT('',#40043);
#11521=VERTEX_POINT('',#40046);
#11522=VERTEX_POINT('',#40052);
#11523=VERTEX_POINT('',#40056);
#11524=VERTEX_POINT('',#40060);
#11525=VERTEX_POINT('',#40063);
#14048=EDGE_CURVE('',#11337,#11337,#5919,.T.);
#14049=EDGE_CURVE('',#11337,#11338,#7064,.T.);
#14050=EDGE_CURVE('',#11338,#11339,#5920,.T.);
#14051=EDGE_CURVE('',#11339,#11338,#5921,.T.);
#14052=EDGE_CURVE('',#11339,#11340,#7065,.T.);
#14053=EDGE_CURVE('',#11340,#11340,#5922,.T.);
#14054=EDGE_CURVE('',#11341,#11341,#5923,.T.);
#14055=EDGE_CURVE('',#11342,#11343,#7066,.T.);
#14056=EDGE_CURVE('',#11342,#11344,#7067,.T.);
#14057=EDGE_CURVE('',#11344,#11345,#7068,.T.);
#14058=EDGE_CURVE('',#11343,#11345,#7069,.T.);
#14059=EDGE_CURVE('',#11343,#11346,#5924,.T.);
#14060=EDGE_CURVE('',#11345,#11347,#7070,.T.);
#14061=EDGE_CURVE('',#11346,#11347,#7071,.T.);
#14062=EDGE_CURVE('',#11346,#11348,#7072,.T.);
#14063=EDGE_CURVE('',#11347,#11349,#7073,.T.);
#14064=EDGE_CURVE('',#11348,#11349,#7074,.T.);
#14065=EDGE_CURVE('',#11348,#11342,#5925,.T.);
#14066=EDGE_CURVE('',#11349,#11344,#7075,.T.);
#14067=EDGE_CURVE('',#11350,#11351,#7076,.T.);
#14068=EDGE_CURVE('',#11350,#11352,#7077,.T.);
#14069=EDGE_CURVE('',#11352,#11353,#7078,.T.);
#14070=EDGE_CURVE('',#11351,#11353,#7079,.T.);
#14071=EDGE_CURVE('',#11351,#11354,#5926,.T.);
#14072=EDGE_CURVE('',#11353,#11355,#7080,.T.);
#14073=EDGE_CURVE('',#11354,#11355,#7081,.T.);
#14074=EDGE_CURVE('',#11354,#11356,#7082,.T.);
#14075=EDGE_CURVE('',#11355,#11357,#7083,.T.);
#14076=EDGE_CURVE('',#11356,#11357,#7084,.T.);
#14077=EDGE_CURVE('',#11356,#11350,#5927,.T.);
#14078=EDGE_CURVE('',#11357,#11352,#7085,.T.);
#14079=EDGE_CURVE('',#11358,#11359,#7086,.T.);
#14080=EDGE_CURVE('',#11358,#11360,#7087,.T.);
#14081=EDGE_CURVE('',#11360,#11361,#7088,.T.);
#14082=EDGE_CURVE('',#11359,#11361,#7089,.T.);
#14083=EDGE_CURVE('',#11359,#11362,#5928,.T.);
#14084=EDGE_CURVE('',#11361,#11363,#7090,.T.);
#14085=EDGE_CURVE('',#11362,#11363,#7091,.T.);
#14086=EDGE_CURVE('',#11362,#11364,#7092,.T.);
#14087=EDGE_CURVE('',#11363,#11365,#7093,.T.);
#14088=EDGE_CURVE('',#11364,#11365,#7094,.T.);
#14089=EDGE_CURVE('',#11364,#11358,#5929,.T.);
#14090=EDGE_CURVE('',#11365,#11360,#7095,.T.);
#14091=EDGE_CURVE('',#11366,#11367,#7096,.T.);
#14092=EDGE_CURVE('',#11366,#11368,#7097,.T.);
#14093=EDGE_CURVE('',#11368,#11369,#7098,.T.);
#14094=EDGE_CURVE('',#11367,#11369,#7099,.T.);
#14095=EDGE_CURVE('',#11367,#11370,#5930,.T.);
#14096=EDGE_CURVE('',#11369,#11371,#7100,.T.);
#14097=EDGE_CURVE('',#11370,#11371,#7101,.T.);
#14098=EDGE_CURVE('',#11370,#11372,#7102,.T.);
#14099=EDGE_CURVE('',#11371,#11373,#7103,.T.);
#14100=EDGE_CURVE('',#11372,#11373,#7104,.T.);
#14101=EDGE_CURVE('',#11372,#11366,#5931,.T.);
#14102=EDGE_CURVE('',#11373,#11368,#7105,.T.);
#14103=EDGE_CURVE('',#11374,#11375,#7106,.T.);
#14104=EDGE_CURVE('',#11374,#11376,#7107,.T.);
#14105=EDGE_CURVE('',#11376,#11377,#7108,.T.);
#14106=EDGE_CURVE('',#11375,#11377,#7109,.T.);
#14107=EDGE_CURVE('',#11375,#11378,#5932,.T.);
#14108=EDGE_CURVE('',#11377,#11379,#7110,.T.);
#14109=EDGE_CURVE('',#11378,#11379,#7111,.T.);
#14110=EDGE_CURVE('',#11378,#11380,#7112,.T.);
#14111=EDGE_CURVE('',#11379,#11381,#7113,.T.);
#14112=EDGE_CURVE('',#11380,#11381,#7114,.T.);
#14113=EDGE_CURVE('',#11380,#11374,#5933,.T.);
#14114=EDGE_CURVE('',#11381,#11376,#7115,.T.);
#14115=EDGE_CURVE('',#11382,#11383,#7116,.T.);
#14116=EDGE_CURVE('',#11382,#11384,#7117,.T.);
#14117=EDGE_CURVE('',#11384,#11385,#7118,.T.);
#14118=EDGE_CURVE('',#11383,#11385,#7119,.T.);
#14119=EDGE_CURVE('',#11383,#11386,#5934,.T.);
#14120=EDGE_CURVE('',#11385,#11387,#7120,.T.);
#14121=EDGE_CURVE('',#11386,#11387,#7121,.T.);
#14122=EDGE_CURVE('',#11386,#11388,#7122,.T.);
#14123=EDGE_CURVE('',#11387,#11389,#7123,.T.);
#14124=EDGE_CURVE('',#11388,#11389,#7124,.T.);
#14125=EDGE_CURVE('',#11388,#11382,#5935,.T.);
#14126=EDGE_CURVE('',#11389,#11384,#7125,.T.);
#14127=EDGE_CURVE('',#11390,#11391,#7126,.T.);
#14128=EDGE_CURVE('',#11390,#11392,#7127,.T.);
#14129=EDGE_CURVE('',#11392,#11393,#7128,.T.);
#14130=EDGE_CURVE('',#11391,#11393,#7129,.T.);
#14131=EDGE_CURVE('',#11391,#11394,#5936,.T.);
#14132=EDGE_CURVE('',#11393,#11395,#7130,.T.);
#14133=EDGE_CURVE('',#11394,#11395,#7131,.T.);
#14134=EDGE_CURVE('',#11394,#11396,#7132,.T.);
#14135=EDGE_CURVE('',#11395,#11397,#7133,.T.);
#14136=EDGE_CURVE('',#11396,#11397,#7134,.T.);
#14137=EDGE_CURVE('',#11396,#11390,#5937,.T.);
#14138=EDGE_CURVE('',#11397,#11392,#7135,.T.);
#14139=EDGE_CURVE('',#11398,#11399,#7136,.T.);
#14140=EDGE_CURVE('',#11398,#11400,#7137,.T.);
#14141=EDGE_CURVE('',#11400,#11401,#7138,.T.);
#14142=EDGE_CURVE('',#11399,#11401,#7139,.T.);
#14143=EDGE_CURVE('',#11399,#11402,#5938,.T.);
#14144=EDGE_CURVE('',#11401,#11403,#7140,.T.);
#14145=EDGE_CURVE('',#11402,#11403,#7141,.T.);
#14146=EDGE_CURVE('',#11402,#11404,#7142,.T.);
#14147=EDGE_CURVE('',#11403,#11405,#7143,.T.);
#14148=EDGE_CURVE('',#11404,#11405,#7144,.T.);
#14149=EDGE_CURVE('',#11404,#11398,#5939,.T.);
#14150=EDGE_CURVE('',#11405,#11400,#7145,.T.);
#14151=EDGE_CURVE('',#11406,#11407,#7146,.T.);
#14152=EDGE_CURVE('',#11406,#11408,#7147,.T.);
#14153=EDGE_CURVE('',#11408,#11409,#7148,.T.);
#14154=EDGE_CURVE('',#11407,#11409,#7149,.T.);
#14155=EDGE_CURVE('',#11407,#11410,#5940,.T.);
#14156=EDGE_CURVE('',#11409,#11411,#7150,.T.);
#14157=EDGE_CURVE('',#11410,#11411,#7151,.T.);
#14158=EDGE_CURVE('',#11410,#11412,#7152,.T.);
#14159=EDGE_CURVE('',#11411,#11413,#7153,.T.);
#14160=EDGE_CURVE('',#11412,#11413,#7154,.T.);
#14161=EDGE_CURVE('',#11412,#11406,#5941,.T.);
#14162=EDGE_CURVE('',#11413,#11408,#7155,.T.);
#14163=EDGE_CURVE('',#11414,#11415,#7156,.T.);
#14164=EDGE_CURVE('',#11414,#11416,#7157,.T.);
#14165=EDGE_CURVE('',#11416,#11417,#7158,.T.);
#14166=EDGE_CURVE('',#11415,#11417,#7159,.T.);
#14167=EDGE_CURVE('',#11415,#11418,#5942,.T.);
#14168=EDGE_CURVE('',#11417,#11419,#7160,.T.);
#14169=EDGE_CURVE('',#11418,#11419,#7161,.T.);
#14170=EDGE_CURVE('',#11418,#11420,#7162,.T.);
#14171=EDGE_CURVE('',#11419,#11421,#7163,.T.);
#14172=EDGE_CURVE('',#11420,#11421,#7164,.T.);
#14173=EDGE_CURVE('',#11420,#11414,#5943,.T.);
#14174=EDGE_CURVE('',#11421,#11416,#7165,.T.);
#14175=EDGE_CURVE('',#11422,#11423,#7166,.T.);
#14176=EDGE_CURVE('',#11422,#11424,#7167,.T.);
#14177=EDGE_CURVE('',#11424,#11425,#7168,.T.);
#14178=EDGE_CURVE('',#11423,#11425,#7169,.T.);
#14179=EDGE_CURVE('',#11423,#11426,#5944,.T.);
#14180=EDGE_CURVE('',#11425,#11427,#7170,.T.);
#14181=EDGE_CURVE('',#11426,#11427,#7171,.T.);
#14182=EDGE_CURVE('',#11426,#11428,#7172,.T.);
#14183=EDGE_CURVE('',#11427,#11429,#7173,.T.);
#14184=EDGE_CURVE('',#11428,#11429,#7174,.T.);
#14185=EDGE_CURVE('',#11428,#11422,#5945,.T.);
#14186=EDGE_CURVE('',#11429,#11424,#7175,.T.);
#14187=EDGE_CURVE('',#11430,#11431,#7176,.T.);
#14188=EDGE_CURVE('',#11430,#11432,#7177,.T.);
#14189=EDGE_CURVE('',#11432,#11433,#7178,.T.);
#14190=EDGE_CURVE('',#11431,#11433,#7179,.T.);
#14191=EDGE_CURVE('',#11431,#11434,#5946,.T.);
#14192=EDGE_CURVE('',#11433,#11435,#7180,.T.);
#14193=EDGE_CURVE('',#11434,#11435,#7181,.T.);
#14194=EDGE_CURVE('',#11434,#11436,#7182,.T.);
#14195=EDGE_CURVE('',#11435,#11437,#7183,.T.);
#14196=EDGE_CURVE('',#11436,#11437,#7184,.T.);
#14197=EDGE_CURVE('',#11436,#11430,#5947,.T.);
#14198=EDGE_CURVE('',#11437,#11432,#7185,.T.);
#14199=EDGE_CURVE('',#11438,#11439,#7186,.T.);
#14200=EDGE_CURVE('',#11438,#11440,#7187,.T.);
#14201=EDGE_CURVE('',#11440,#11441,#7188,.T.);
#14202=EDGE_CURVE('',#11439,#11441,#7189,.T.);
#14203=EDGE_CURVE('',#11439,#11442,#5948,.T.);
#14204=EDGE_CURVE('',#11441,#11443,#7190,.T.);
#14205=EDGE_CURVE('',#11442,#11443,#7191,.T.);
#14206=EDGE_CURVE('',#11442,#11444,#7192,.T.);
#14207=EDGE_CURVE('',#11443,#11445,#7193,.T.);
#14208=EDGE_CURVE('',#11444,#11445,#7194,.T.);
#14209=EDGE_CURVE('',#11444,#11438,#5949,.T.);
#14210=EDGE_CURVE('',#11445,#11440,#7195,.T.);
#14211=EDGE_CURVE('',#11446,#11447,#7196,.T.);
#14212=EDGE_CURVE('',#11446,#11448,#7197,.T.);
#14213=EDGE_CURVE('',#11448,#11449,#7198,.T.);
#14214=EDGE_CURVE('',#11447,#11449,#7199,.T.);
#14215=EDGE_CURVE('',#11447,#11450,#5950,.T.);
#14216=EDGE_CURVE('',#11449,#11451,#7200,.T.);
#14217=EDGE_CURVE('',#11450,#11451,#7201,.T.);
#14218=EDGE_CURVE('',#11450,#11452,#7202,.T.);
#14219=EDGE_CURVE('',#11451,#11453,#7203,.T.);
#14220=EDGE_CURVE('',#11452,#11453,#7204,.T.);
#14221=EDGE_CURVE('',#11452,#11446,#5951,.T.);
#14222=EDGE_CURVE('',#11453,#11448,#7205,.T.);
#14223=EDGE_CURVE('',#11454,#11455,#7206,.T.);
#14224=EDGE_CURVE('',#11454,#11456,#7207,.T.);
#14225=EDGE_CURVE('',#11456,#11457,#7208,.T.);
#14226=EDGE_CURVE('',#11455,#11457,#7209,.T.);
#14227=EDGE_CURVE('',#11455,#11458,#5952,.T.);
#14228=EDGE_CURVE('',#11457,#11459,#7210,.T.);
#14229=EDGE_CURVE('',#11458,#11459,#7211,.T.);
#14230=EDGE_CURVE('',#11458,#11460,#7212,.T.);
#14231=EDGE_CURVE('',#11459,#11461,#7213,.T.);
#14232=EDGE_CURVE('',#11460,#11461,#7214,.T.);
#14233=EDGE_CURVE('',#11460,#11454,#5953,.T.);
#14234=EDGE_CURVE('',#11461,#11456,#7215,.T.);
#14235=EDGE_CURVE('',#11462,#11463,#7216,.T.);
#14236=EDGE_CURVE('',#11462,#11464,#7217,.T.);
#14237=EDGE_CURVE('',#11464,#11465,#7218,.T.);
#14238=EDGE_CURVE('',#11463,#11465,#7219,.T.);
#14239=EDGE_CURVE('',#11463,#11466,#5954,.T.);
#14240=EDGE_CURVE('',#11465,#11467,#7220,.T.);
#14241=EDGE_CURVE('',#11466,#11467,#7221,.T.);
#14242=EDGE_CURVE('',#11466,#11468,#7222,.T.);
#14243=EDGE_CURVE('',#11467,#11469,#7223,.T.);
#14244=EDGE_CURVE('',#11468,#11469,#7224,.T.);
#14245=EDGE_CURVE('',#11468,#11462,#5955,.T.);
#14246=EDGE_CURVE('',#11469,#11464,#7225,.T.);
#14247=EDGE_CURVE('',#11470,#11471,#7226,.T.);
#14248=EDGE_CURVE('',#11470,#11472,#7227,.T.);
#14249=EDGE_CURVE('',#11472,#11473,#7228,.T.);
#14250=EDGE_CURVE('',#11471,#11473,#7229,.T.);
#14251=EDGE_CURVE('',#11471,#11474,#5956,.T.);
#14252=EDGE_CURVE('',#11473,#11475,#7230,.T.);
#14253=EDGE_CURVE('',#11474,#11475,#7231,.T.);
#14254=EDGE_CURVE('',#11474,#11476,#7232,.T.);
#14255=EDGE_CURVE('',#11475,#11477,#7233,.T.);
#14256=EDGE_CURVE('',#11476,#11477,#7234,.T.);
#14257=EDGE_CURVE('',#11476,#11470,#5957,.T.);
#14258=EDGE_CURVE('',#11477,#11472,#7235,.T.);
#14259=EDGE_CURVE('',#11478,#11479,#7236,.T.);
#14260=EDGE_CURVE('',#11478,#11480,#7237,.T.);
#14261=EDGE_CURVE('',#11480,#11481,#7238,.T.);
#14262=EDGE_CURVE('',#11479,#11481,#7239,.T.);
#14263=EDGE_CURVE('',#11479,#11482,#5958,.T.);
#14264=EDGE_CURVE('',#11481,#11483,#7240,.T.);
#14265=EDGE_CURVE('',#11482,#11483,#7241,.T.);
#14266=EDGE_CURVE('',#11482,#11484,#7242,.T.);
#14267=EDGE_CURVE('',#11483,#11485,#7243,.T.);
#14268=EDGE_CURVE('',#11484,#11485,#7244,.T.);
#14269=EDGE_CURVE('',#11484,#11478,#5959,.T.);
#14270=EDGE_CURVE('',#11485,#11480,#7245,.T.);
#14271=EDGE_CURVE('',#11486,#11487,#7246,.T.);
#14272=EDGE_CURVE('',#11486,#11488,#7247,.T.);
#14273=EDGE_CURVE('',#11488,#11489,#7248,.T.);
#14274=EDGE_CURVE('',#11487,#11489,#7249,.T.);
#14275=EDGE_CURVE('',#11487,#11490,#5960,.T.);
#14276=EDGE_CURVE('',#11489,#11491,#7250,.T.);
#14277=EDGE_CURVE('',#11490,#11491,#7251,.T.);
#14278=EDGE_CURVE('',#11490,#11492,#7252,.T.);
#14279=EDGE_CURVE('',#11491,#11493,#7253,.T.);
#14280=EDGE_CURVE('',#11492,#11493,#7254,.T.);
#14281=EDGE_CURVE('',#11492,#11486,#5961,.T.);
#14282=EDGE_CURVE('',#11493,#11488,#7255,.T.);
#14283=EDGE_CURVE('',#11494,#11495,#7256,.T.);
#14284=EDGE_CURVE('',#11494,#11496,#7257,.T.);
#14285=EDGE_CURVE('',#11496,#11497,#7258,.T.);
#14286=EDGE_CURVE('',#11495,#11497,#7259,.T.);
#14287=EDGE_CURVE('',#11495,#11498,#5962,.T.);
#14288=EDGE_CURVE('',#11497,#11499,#7260,.T.);
#14289=EDGE_CURVE('',#11498,#11499,#7261,.T.);
#14290=EDGE_CURVE('',#11498,#11500,#7262,.T.);
#14291=EDGE_CURVE('',#11499,#11501,#7263,.T.);
#14292=EDGE_CURVE('',#11500,#11501,#7264,.T.);
#14293=EDGE_CURVE('',#11500,#11494,#5963,.T.);
#14294=EDGE_CURVE('',#11501,#11496,#7265,.T.);
#14295=EDGE_CURVE('',#11502,#11503,#7266,.T.);
#14296=EDGE_CURVE('',#11502,#11504,#7267,.T.);
#14297=EDGE_CURVE('',#11504,#11505,#7268,.T.);
#14298=EDGE_CURVE('',#11503,#11505,#7269,.T.);
#14299=EDGE_CURVE('',#11503,#11506,#5964,.T.);
#14300=EDGE_CURVE('',#11505,#11507,#7270,.T.);
#14301=EDGE_CURVE('',#11506,#11507,#7271,.T.);
#14302=EDGE_CURVE('',#11506,#11508,#7272,.T.);
#14303=EDGE_CURVE('',#11507,#11509,#7273,.T.);
#14304=EDGE_CURVE('',#11508,#11509,#7274,.T.);
#14305=EDGE_CURVE('',#11508,#11502,#5965,.T.);
#14306=EDGE_CURVE('',#11509,#11504,#7275,.T.);
#14307=EDGE_CURVE('',#11510,#11511,#7276,.T.);
#14308=EDGE_CURVE('',#11512,#11510,#7277,.T.);
#14309=EDGE_CURVE('',#11512,#11513,#7278,.T.);
#14310=EDGE_CURVE('',#11513,#11511,#7279,.T.);
#14311=EDGE_CURVE('',#11511,#11514,#237,.T.);
#14312=EDGE_CURVE('',#11513,#11515,#5966,.T.);
#14313=EDGE_CURVE('',#11515,#11514,#7280,.T.);
#14314=EDGE_CURVE('',#11514,#11516,#7281,.T.);
#14315=EDGE_CURVE('',#11515,#11517,#7282,.T.);
#14316=EDGE_CURVE('',#11517,#11516,#7283,.T.);
#14317=EDGE_CURVE('',#11516,#11510,#238,.T.);
#14318=EDGE_CURVE('',#11517,#11512,#5967,.T.);
#14319=EDGE_CURVE('',#11518,#11518,#5968,.T.);
#14320=EDGE_CURVE('',#11518,#11519,#7284,.T.);
#14321=EDGE_CURVE('',#11519,#11519,#5969,.T.);
#14322=EDGE_CURVE('',#11520,#11520,#5970,.T.);
#14323=EDGE_CURVE('',#11521,#11521,#5971,.T.);
#14324=EDGE_CURVE('',#11521,#11520,#7285,.T.);
#14325=EDGE_CURVE('',#11340,#11521,#7286,.T.);
#14326=EDGE_CURVE('',#11341,#11522,#7287,.T.);
#14327=EDGE_CURVE('',#11522,#11522,#5972,.T.);
#14328=EDGE_CURVE('',#11522,#11523,#7288,.T.);
#14329=EDGE_CURVE('',#11523,#11523,#5973,.T.);
#14330=EDGE_CURVE('',#11524,#11524,#5974,.T.);
#14331=EDGE_CURVE('',#11524,#11525,#7289,.T.);
#14332=EDGE_CURVE('',#11525,#11525,#5975,.T.);
#18651=ORIENTED_EDGE('',*,*,#14048,.T.);
#18652=ORIENTED_EDGE('',*,*,#14049,.T.);
#18653=ORIENTED_EDGE('',*,*,#14050,.T.);
#18654=ORIENTED_EDGE('',*,*,#14051,.T.);
#18655=ORIENTED_EDGE('',*,*,#14049,.F.);
#18656=ORIENTED_EDGE('',*,*,#14050,.F.);
#18657=ORIENTED_EDGE('',*,*,#14051,.F.);
#18658=ORIENTED_EDGE('',*,*,#14052,.T.);
#18659=ORIENTED_EDGE('',*,*,#14053,.T.);
#18660=ORIENTED_EDGE('',*,*,#14052,.F.);
#18661=ORIENTED_EDGE('',*,*,#14048,.F.);
#18662=ORIENTED_EDGE('',*,*,#14054,.F.);
#18663=ORIENTED_EDGE('',*,*,#14055,.F.);
#18664=ORIENTED_EDGE('',*,*,#14056,.T.);
#18665=ORIENTED_EDGE('',*,*,#14057,.T.);
#18666=ORIENTED_EDGE('',*,*,#14058,.F.);
#18667=ORIENTED_EDGE('',*,*,#14059,.F.);
#18668=ORIENTED_EDGE('',*,*,#14058,.T.);
#18669=ORIENTED_EDGE('',*,*,#14060,.T.);
#18670=ORIENTED_EDGE('',*,*,#14061,.F.);
#18671=ORIENTED_EDGE('',*,*,#14062,.F.);
#18672=ORIENTED_EDGE('',*,*,#14061,.T.);
#18673=ORIENTED_EDGE('',*,*,#14063,.T.);
#18674=ORIENTED_EDGE('',*,*,#14064,.F.);
#18675=ORIENTED_EDGE('',*,*,#14065,.F.);
#18676=ORIENTED_EDGE('',*,*,#14064,.T.);
#18677=ORIENTED_EDGE('',*,*,#14066,.T.);
#18678=ORIENTED_EDGE('',*,*,#14056,.F.);
#18679=ORIENTED_EDGE('',*,*,#14066,.F.);
#18680=ORIENTED_EDGE('',*,*,#14063,.F.);
#18681=ORIENTED_EDGE('',*,*,#14060,.F.);
#18682=ORIENTED_EDGE('',*,*,#14057,.F.);
#18683=ORIENTED_EDGE('',*,*,#14067,.F.);
#18684=ORIENTED_EDGE('',*,*,#14068,.T.);
#18685=ORIENTED_EDGE('',*,*,#14069,.T.);
#18686=ORIENTED_EDGE('',*,*,#14070,.F.);
#18687=ORIENTED_EDGE('',*,*,#14071,.F.);
#18688=ORIENTED_EDGE('',*,*,#14070,.T.);
#18689=ORIENTED_EDGE('',*,*,#14072,.T.);
#18690=ORIENTED_EDGE('',*,*,#14073,.F.);
#18691=ORIENTED_EDGE('',*,*,#14074,.F.);
#18692=ORIENTED_EDGE('',*,*,#14073,.T.);
#18693=ORIENTED_EDGE('',*,*,#14075,.T.);
#18694=ORIENTED_EDGE('',*,*,#14076,.F.);
#18695=ORIENTED_EDGE('',*,*,#14077,.F.);
#18696=ORIENTED_EDGE('',*,*,#14076,.T.);
#18697=ORIENTED_EDGE('',*,*,#14078,.T.);
#18698=ORIENTED_EDGE('',*,*,#14068,.F.);
#18699=ORIENTED_EDGE('',*,*,#14078,.F.);
#18700=ORIENTED_EDGE('',*,*,#14075,.F.);
#18701=ORIENTED_EDGE('',*,*,#14072,.F.);
#18702=ORIENTED_EDGE('',*,*,#14069,.F.);
#18703=ORIENTED_EDGE('',*,*,#14079,.F.);
#18704=ORIENTED_EDGE('',*,*,#14080,.T.);
#18705=ORIENTED_EDGE('',*,*,#14081,.T.);
#18706=ORIENTED_EDGE('',*,*,#14082,.F.);
#18707=ORIENTED_EDGE('',*,*,#14083,.F.);
#18708=ORIENTED_EDGE('',*,*,#14082,.T.);
#18709=ORIENTED_EDGE('',*,*,#14084,.T.);
#18710=ORIENTED_EDGE('',*,*,#14085,.F.);
#18711=ORIENTED_EDGE('',*,*,#14086,.F.);
#18712=ORIENTED_EDGE('',*,*,#14085,.T.);
#18713=ORIENTED_EDGE('',*,*,#14087,.T.);
#18714=ORIENTED_EDGE('',*,*,#14088,.F.);
#18715=ORIENTED_EDGE('',*,*,#14089,.F.);
#18716=ORIENTED_EDGE('',*,*,#14088,.T.);
#18717=ORIENTED_EDGE('',*,*,#14090,.T.);
#18718=ORIENTED_EDGE('',*,*,#14080,.F.);
#18719=ORIENTED_EDGE('',*,*,#14090,.F.);
#18720=ORIENTED_EDGE('',*,*,#14087,.F.);
#18721=ORIENTED_EDGE('',*,*,#14084,.F.);
#18722=ORIENTED_EDGE('',*,*,#14081,.F.);
#18723=ORIENTED_EDGE('',*,*,#14091,.F.);
#18724=ORIENTED_EDGE('',*,*,#14092,.T.);
#18725=ORIENTED_EDGE('',*,*,#14093,.T.);
#18726=ORIENTED_EDGE('',*,*,#14094,.F.);
#18727=ORIENTED_EDGE('',*,*,#14095,.F.);
#18728=ORIENTED_EDGE('',*,*,#14094,.T.);
#18729=ORIENTED_EDGE('',*,*,#14096,.T.);
#18730=ORIENTED_EDGE('',*,*,#14097,.F.);
#18731=ORIENTED_EDGE('',*,*,#14098,.F.);
#18732=ORIENTED_EDGE('',*,*,#14097,.T.);
#18733=ORIENTED_EDGE('',*,*,#14099,.T.);
#18734=ORIENTED_EDGE('',*,*,#14100,.F.);
#18735=ORIENTED_EDGE('',*,*,#14101,.F.);
#18736=ORIENTED_EDGE('',*,*,#14100,.T.);
#18737=ORIENTED_EDGE('',*,*,#14102,.T.);
#18738=ORIENTED_EDGE('',*,*,#14092,.F.);
#18739=ORIENTED_EDGE('',*,*,#14102,.F.);
#18740=ORIENTED_EDGE('',*,*,#14099,.F.);
#18741=ORIENTED_EDGE('',*,*,#14096,.F.);
#18742=ORIENTED_EDGE('',*,*,#14093,.F.);
#18743=ORIENTED_EDGE('',*,*,#14103,.F.);
#18744=ORIENTED_EDGE('',*,*,#14104,.T.);
#18745=ORIENTED_EDGE('',*,*,#14105,.T.);
#18746=ORIENTED_EDGE('',*,*,#14106,.F.);
#18747=ORIENTED_EDGE('',*,*,#14107,.F.);
#18748=ORIENTED_EDGE('',*,*,#14106,.T.);
#18749=ORIENTED_EDGE('',*,*,#14108,.T.);
#18750=ORIENTED_EDGE('',*,*,#14109,.F.);
#18751=ORIENTED_EDGE('',*,*,#14110,.F.);
#18752=ORIENTED_EDGE('',*,*,#14109,.T.);
#18753=ORIENTED_EDGE('',*,*,#14111,.T.);
#18754=ORIENTED_EDGE('',*,*,#14112,.F.);
#18755=ORIENTED_EDGE('',*,*,#14113,.F.);
#18756=ORIENTED_EDGE('',*,*,#14112,.T.);
#18757=ORIENTED_EDGE('',*,*,#14114,.T.);
#18758=ORIENTED_EDGE('',*,*,#14104,.F.);
#18759=ORIENTED_EDGE('',*,*,#14114,.F.);
#18760=ORIENTED_EDGE('',*,*,#14111,.F.);
#18761=ORIENTED_EDGE('',*,*,#14108,.F.);
#18762=ORIENTED_EDGE('',*,*,#14105,.F.);
#18763=ORIENTED_EDGE('',*,*,#14115,.F.);
#18764=ORIENTED_EDGE('',*,*,#14116,.T.);
#18765=ORIENTED_EDGE('',*,*,#14117,.T.);
#18766=ORIENTED_EDGE('',*,*,#14118,.F.);
#18767=ORIENTED_EDGE('',*,*,#14119,.F.);
#18768=ORIENTED_EDGE('',*,*,#14118,.T.);
#18769=ORIENTED_EDGE('',*,*,#14120,.T.);
#18770=ORIENTED_EDGE('',*,*,#14121,.F.);
#18771=ORIENTED_EDGE('',*,*,#14122,.F.);
#18772=ORIENTED_EDGE('',*,*,#14121,.T.);
#18773=ORIENTED_EDGE('',*,*,#14123,.T.);
#18774=ORIENTED_EDGE('',*,*,#14124,.F.);
#18775=ORIENTED_EDGE('',*,*,#14125,.F.);
#18776=ORIENTED_EDGE('',*,*,#14124,.T.);
#18777=ORIENTED_EDGE('',*,*,#14126,.T.);
#18778=ORIENTED_EDGE('',*,*,#14116,.F.);
#18779=ORIENTED_EDGE('',*,*,#14126,.F.);
#18780=ORIENTED_EDGE('',*,*,#14123,.F.);
#18781=ORIENTED_EDGE('',*,*,#14120,.F.);
#18782=ORIENTED_EDGE('',*,*,#14117,.F.);
#18783=ORIENTED_EDGE('',*,*,#14127,.F.);
#18784=ORIENTED_EDGE('',*,*,#14128,.T.);
#18785=ORIENTED_EDGE('',*,*,#14129,.T.);
#18786=ORIENTED_EDGE('',*,*,#14130,.F.);
#18787=ORIENTED_EDGE('',*,*,#14131,.F.);
#18788=ORIENTED_EDGE('',*,*,#14130,.T.);
#18789=ORIENTED_EDGE('',*,*,#14132,.T.);
#18790=ORIENTED_EDGE('',*,*,#14133,.F.);
#18791=ORIENTED_EDGE('',*,*,#14134,.F.);
#18792=ORIENTED_EDGE('',*,*,#14133,.T.);
#18793=ORIENTED_EDGE('',*,*,#14135,.T.);
#18794=ORIENTED_EDGE('',*,*,#14136,.F.);
#18795=ORIENTED_EDGE('',*,*,#14137,.F.);
#18796=ORIENTED_EDGE('',*,*,#14136,.T.);
#18797=ORIENTED_EDGE('',*,*,#14138,.T.);
#18798=ORIENTED_EDGE('',*,*,#14128,.F.);
#18799=ORIENTED_EDGE('',*,*,#14138,.F.);
#18800=ORIENTED_EDGE('',*,*,#14135,.F.);
#18801=ORIENTED_EDGE('',*,*,#14132,.F.);
#18802=ORIENTED_EDGE('',*,*,#14129,.F.);
#18803=ORIENTED_EDGE('',*,*,#14139,.F.);
#18804=ORIENTED_EDGE('',*,*,#14140,.T.);
#18805=ORIENTED_EDGE('',*,*,#14141,.T.);
#18806=ORIENTED_EDGE('',*,*,#14142,.F.);
#18807=ORIENTED_EDGE('',*,*,#14143,.F.);
#18808=ORIENTED_EDGE('',*,*,#14142,.T.);
#18809=ORIENTED_EDGE('',*,*,#14144,.T.);
#18810=ORIENTED_EDGE('',*,*,#14145,.F.);
#18811=ORIENTED_EDGE('',*,*,#14146,.F.);
#18812=ORIENTED_EDGE('',*,*,#14145,.T.);
#18813=ORIENTED_EDGE('',*,*,#14147,.T.);
#18814=ORIENTED_EDGE('',*,*,#14148,.F.);
#18815=ORIENTED_EDGE('',*,*,#14149,.F.);
#18816=ORIENTED_EDGE('',*,*,#14148,.T.);
#18817=ORIENTED_EDGE('',*,*,#14150,.T.);
#18818=ORIENTED_EDGE('',*,*,#14140,.F.);
#18819=ORIENTED_EDGE('',*,*,#14150,.F.);
#18820=ORIENTED_EDGE('',*,*,#14147,.F.);
#18821=ORIENTED_EDGE('',*,*,#14144,.F.);
#18822=ORIENTED_EDGE('',*,*,#14141,.F.);
#18823=ORIENTED_EDGE('',*,*,#14151,.F.);
#18824=ORIENTED_EDGE('',*,*,#14152,.T.);
#18825=ORIENTED_EDGE('',*,*,#14153,.T.);
#18826=ORIENTED_EDGE('',*,*,#14154,.F.);
#18827=ORIENTED_EDGE('',*,*,#14155,.F.);
#18828=ORIENTED_EDGE('',*,*,#14154,.T.);
#18829=ORIENTED_EDGE('',*,*,#14156,.T.);
#18830=ORIENTED_EDGE('',*,*,#14157,.F.);
#18831=ORIENTED_EDGE('',*,*,#14158,.F.);
#18832=ORIENTED_EDGE('',*,*,#14157,.T.);
#18833=ORIENTED_EDGE('',*,*,#14159,.T.);
#18834=ORIENTED_EDGE('',*,*,#14160,.F.);
#18835=ORIENTED_EDGE('',*,*,#14161,.F.);
#18836=ORIENTED_EDGE('',*,*,#14160,.T.);
#18837=ORIENTED_EDGE('',*,*,#14162,.T.);
#18838=ORIENTED_EDGE('',*,*,#14152,.F.);
#18839=ORIENTED_EDGE('',*,*,#14162,.F.);
#18840=ORIENTED_EDGE('',*,*,#14159,.F.);
#18841=ORIENTED_EDGE('',*,*,#14156,.F.);
#18842=ORIENTED_EDGE('',*,*,#14153,.F.);
#18843=ORIENTED_EDGE('',*,*,#14163,.F.);
#18844=ORIENTED_EDGE('',*,*,#14164,.T.);
#18845=ORIENTED_EDGE('',*,*,#14165,.T.);
#18846=ORIENTED_EDGE('',*,*,#14166,.F.);
#18847=ORIENTED_EDGE('',*,*,#14167,.F.);
#18848=ORIENTED_EDGE('',*,*,#14166,.T.);
#18849=ORIENTED_EDGE('',*,*,#14168,.T.);
#18850=ORIENTED_EDGE('',*,*,#14169,.F.);
#18851=ORIENTED_EDGE('',*,*,#14170,.F.);
#18852=ORIENTED_EDGE('',*,*,#14169,.T.);
#18853=ORIENTED_EDGE('',*,*,#14171,.T.);
#18854=ORIENTED_EDGE('',*,*,#14172,.F.);
#18855=ORIENTED_EDGE('',*,*,#14173,.F.);
#18856=ORIENTED_EDGE('',*,*,#14172,.T.);
#18857=ORIENTED_EDGE('',*,*,#14174,.T.);
#18858=ORIENTED_EDGE('',*,*,#14164,.F.);
#18859=ORIENTED_EDGE('',*,*,#14174,.F.);
#18860=ORIENTED_EDGE('',*,*,#14171,.F.);
#18861=ORIENTED_EDGE('',*,*,#14168,.F.);
#18862=ORIENTED_EDGE('',*,*,#14165,.F.);
#18863=ORIENTED_EDGE('',*,*,#14175,.F.);
#18864=ORIENTED_EDGE('',*,*,#14176,.T.);
#18865=ORIENTED_EDGE('',*,*,#14177,.T.);
#18866=ORIENTED_EDGE('',*,*,#14178,.F.);
#18867=ORIENTED_EDGE('',*,*,#14179,.F.);
#18868=ORIENTED_EDGE('',*,*,#14178,.T.);
#18869=ORIENTED_EDGE('',*,*,#14180,.T.);
#18870=ORIENTED_EDGE('',*,*,#14181,.F.);
#18871=ORIENTED_EDGE('',*,*,#14182,.F.);
#18872=ORIENTED_EDGE('',*,*,#14181,.T.);
#18873=ORIENTED_EDGE('',*,*,#14183,.T.);
#18874=ORIENTED_EDGE('',*,*,#14184,.F.);
#18875=ORIENTED_EDGE('',*,*,#14185,.F.);
#18876=ORIENTED_EDGE('',*,*,#14184,.T.);
#18877=ORIENTED_EDGE('',*,*,#14186,.T.);
#18878=ORIENTED_EDGE('',*,*,#14176,.F.);
#18879=ORIENTED_EDGE('',*,*,#14186,.F.);
#18880=ORIENTED_EDGE('',*,*,#14183,.F.);
#18881=ORIENTED_EDGE('',*,*,#14180,.F.);
#18882=ORIENTED_EDGE('',*,*,#14177,.F.);
#18883=ORIENTED_EDGE('',*,*,#14187,.F.);
#18884=ORIENTED_EDGE('',*,*,#14188,.T.);
#18885=ORIENTED_EDGE('',*,*,#14189,.T.);
#18886=ORIENTED_EDGE('',*,*,#14190,.F.);
#18887=ORIENTED_EDGE('',*,*,#14191,.F.);
#18888=ORIENTED_EDGE('',*,*,#14190,.T.);
#18889=ORIENTED_EDGE('',*,*,#14192,.T.);
#18890=ORIENTED_EDGE('',*,*,#14193,.F.);
#18891=ORIENTED_EDGE('',*,*,#14194,.F.);
#18892=ORIENTED_EDGE('',*,*,#14193,.T.);
#18893=ORIENTED_EDGE('',*,*,#14195,.T.);
#18894=ORIENTED_EDGE('',*,*,#14196,.F.);
#18895=ORIENTED_EDGE('',*,*,#14197,.F.);
#18896=ORIENTED_EDGE('',*,*,#14196,.T.);
#18897=ORIENTED_EDGE('',*,*,#14198,.T.);
#18898=ORIENTED_EDGE('',*,*,#14188,.F.);
#18899=ORIENTED_EDGE('',*,*,#14198,.F.);
#18900=ORIENTED_EDGE('',*,*,#14195,.F.);
#18901=ORIENTED_EDGE('',*,*,#14192,.F.);
#18902=ORIENTED_EDGE('',*,*,#14189,.F.);
#18903=ORIENTED_EDGE('',*,*,#14199,.F.);
#18904=ORIENTED_EDGE('',*,*,#14200,.T.);
#18905=ORIENTED_EDGE('',*,*,#14201,.T.);
#18906=ORIENTED_EDGE('',*,*,#14202,.F.);
#18907=ORIENTED_EDGE('',*,*,#14203,.F.);
#18908=ORIENTED_EDGE('',*,*,#14202,.T.);
#18909=ORIENTED_EDGE('',*,*,#14204,.T.);
#18910=ORIENTED_EDGE('',*,*,#14205,.F.);
#18911=ORIENTED_EDGE('',*,*,#14206,.F.);
#18912=ORIENTED_EDGE('',*,*,#14205,.T.);
#18913=ORIENTED_EDGE('',*,*,#14207,.T.);
#18914=ORIENTED_EDGE('',*,*,#14208,.F.);
#18915=ORIENTED_EDGE('',*,*,#14209,.F.);
#18916=ORIENTED_EDGE('',*,*,#14208,.T.);
#18917=ORIENTED_EDGE('',*,*,#14210,.T.);
#18918=ORIENTED_EDGE('',*,*,#14200,.F.);
#18919=ORIENTED_EDGE('',*,*,#14210,.F.);
#18920=ORIENTED_EDGE('',*,*,#14207,.F.);
#18921=ORIENTED_EDGE('',*,*,#14204,.F.);
#18922=ORIENTED_EDGE('',*,*,#14201,.F.);
#18923=ORIENTED_EDGE('',*,*,#14211,.F.);
#18924=ORIENTED_EDGE('',*,*,#14212,.T.);
#18925=ORIENTED_EDGE('',*,*,#14213,.T.);
#18926=ORIENTED_EDGE('',*,*,#14214,.F.);
#18927=ORIENTED_EDGE('',*,*,#14215,.F.);
#18928=ORIENTED_EDGE('',*,*,#14214,.T.);
#18929=ORIENTED_EDGE('',*,*,#14216,.T.);
#18930=ORIENTED_EDGE('',*,*,#14217,.F.);
#18931=ORIENTED_EDGE('',*,*,#14218,.F.);
#18932=ORIENTED_EDGE('',*,*,#14217,.T.);
#18933=ORIENTED_EDGE('',*,*,#14219,.T.);
#18934=ORIENTED_EDGE('',*,*,#14220,.F.);
#18935=ORIENTED_EDGE('',*,*,#14221,.F.);
#18936=ORIENTED_EDGE('',*,*,#14220,.T.);
#18937=ORIENTED_EDGE('',*,*,#14222,.T.);
#18938=ORIENTED_EDGE('',*,*,#14212,.F.);
#18939=ORIENTED_EDGE('',*,*,#14222,.F.);
#18940=ORIENTED_EDGE('',*,*,#14219,.F.);
#18941=ORIENTED_EDGE('',*,*,#14216,.F.);
#18942=ORIENTED_EDGE('',*,*,#14213,.F.);
#18943=ORIENTED_EDGE('',*,*,#14223,.F.);
#18944=ORIENTED_EDGE('',*,*,#14224,.T.);
#18945=ORIENTED_EDGE('',*,*,#14225,.T.);
#18946=ORIENTED_EDGE('',*,*,#14226,.F.);
#18947=ORIENTED_EDGE('',*,*,#14227,.F.);
#18948=ORIENTED_EDGE('',*,*,#14226,.T.);
#18949=ORIENTED_EDGE('',*,*,#14228,.T.);
#18950=ORIENTED_EDGE('',*,*,#14229,.F.);
#18951=ORIENTED_EDGE('',*,*,#14230,.F.);
#18952=ORIENTED_EDGE('',*,*,#14229,.T.);
#18953=ORIENTED_EDGE('',*,*,#14231,.T.);
#18954=ORIENTED_EDGE('',*,*,#14232,.F.);
#18955=ORIENTED_EDGE('',*,*,#14233,.F.);
#18956=ORIENTED_EDGE('',*,*,#14232,.T.);
#18957=ORIENTED_EDGE('',*,*,#14234,.T.);
#18958=ORIENTED_EDGE('',*,*,#14224,.F.);
#18959=ORIENTED_EDGE('',*,*,#14234,.F.);
#18960=ORIENTED_EDGE('',*,*,#14231,.F.);
#18961=ORIENTED_EDGE('',*,*,#14228,.F.);
#18962=ORIENTED_EDGE('',*,*,#14225,.F.);
#18963=ORIENTED_EDGE('',*,*,#14235,.F.);
#18964=ORIENTED_EDGE('',*,*,#14236,.T.);
#18965=ORIENTED_EDGE('',*,*,#14237,.T.);
#18966=ORIENTED_EDGE('',*,*,#14238,.F.);
#18967=ORIENTED_EDGE('',*,*,#14239,.F.);
#18968=ORIENTED_EDGE('',*,*,#14238,.T.);
#18969=ORIENTED_EDGE('',*,*,#14240,.T.);
#18970=ORIENTED_EDGE('',*,*,#14241,.F.);
#18971=ORIENTED_EDGE('',*,*,#14242,.F.);
#18972=ORIENTED_EDGE('',*,*,#14241,.T.);
#18973=ORIENTED_EDGE('',*,*,#14243,.T.);
#18974=ORIENTED_EDGE('',*,*,#14244,.F.);
#18975=ORIENTED_EDGE('',*,*,#14245,.F.);
#18976=ORIENTED_EDGE('',*,*,#14244,.T.);
#18977=ORIENTED_EDGE('',*,*,#14246,.T.);
#18978=ORIENTED_EDGE('',*,*,#14236,.F.);
#18979=ORIENTED_EDGE('',*,*,#14246,.F.);
#18980=ORIENTED_EDGE('',*,*,#14243,.F.);
#18981=ORIENTED_EDGE('',*,*,#14240,.F.);
#18982=ORIENTED_EDGE('',*,*,#14237,.F.);
#18983=ORIENTED_EDGE('',*,*,#14247,.F.);
#18984=ORIENTED_EDGE('',*,*,#14248,.T.);
#18985=ORIENTED_EDGE('',*,*,#14249,.T.);
#18986=ORIENTED_EDGE('',*,*,#14250,.F.);
#18987=ORIENTED_EDGE('',*,*,#14251,.F.);
#18988=ORIENTED_EDGE('',*,*,#14250,.T.);
#18989=ORIENTED_EDGE('',*,*,#14252,.T.);
#18990=ORIENTED_EDGE('',*,*,#14253,.F.);
#18991=ORIENTED_EDGE('',*,*,#14254,.F.);
#18992=ORIENTED_EDGE('',*,*,#14253,.T.);
#18993=ORIENTED_EDGE('',*,*,#14255,.T.);
#18994=ORIENTED_EDGE('',*,*,#14256,.F.);
#18995=ORIENTED_EDGE('',*,*,#14257,.F.);
#18996=ORIENTED_EDGE('',*,*,#14256,.T.);
#18997=ORIENTED_EDGE('',*,*,#14258,.T.);
#18998=ORIENTED_EDGE('',*,*,#14248,.F.);
#18999=ORIENTED_EDGE('',*,*,#14258,.F.);
#19000=ORIENTED_EDGE('',*,*,#14255,.F.);
#19001=ORIENTED_EDGE('',*,*,#14252,.F.);
#19002=ORIENTED_EDGE('',*,*,#14249,.F.);
#19003=ORIENTED_EDGE('',*,*,#14259,.F.);
#19004=ORIENTED_EDGE('',*,*,#14260,.T.);
#19005=ORIENTED_EDGE('',*,*,#14261,.T.);
#19006=ORIENTED_EDGE('',*,*,#14262,.F.);
#19007=ORIENTED_EDGE('',*,*,#14263,.F.);
#19008=ORIENTED_EDGE('',*,*,#14262,.T.);
#19009=ORIENTED_EDGE('',*,*,#14264,.T.);
#19010=ORIENTED_EDGE('',*,*,#14265,.F.);
#19011=ORIENTED_EDGE('',*,*,#14266,.F.);
#19012=ORIENTED_EDGE('',*,*,#14265,.T.);
#19013=ORIENTED_EDGE('',*,*,#14267,.T.);
#19014=ORIENTED_EDGE('',*,*,#14268,.F.);
#19015=ORIENTED_EDGE('',*,*,#14269,.F.);
#19016=ORIENTED_EDGE('',*,*,#14268,.T.);
#19017=ORIENTED_EDGE('',*,*,#14270,.T.);
#19018=ORIENTED_EDGE('',*,*,#14260,.F.);
#19019=ORIENTED_EDGE('',*,*,#14270,.F.);
#19020=ORIENTED_EDGE('',*,*,#14267,.F.);
#19021=ORIENTED_EDGE('',*,*,#14264,.F.);
#19022=ORIENTED_EDGE('',*,*,#14261,.F.);
#19023=ORIENTED_EDGE('',*,*,#14271,.F.);
#19024=ORIENTED_EDGE('',*,*,#14272,.T.);
#19025=ORIENTED_EDGE('',*,*,#14273,.T.);
#19026=ORIENTED_EDGE('',*,*,#14274,.F.);
#19027=ORIENTED_EDGE('',*,*,#14275,.F.);
#19028=ORIENTED_EDGE('',*,*,#14274,.T.);
#19029=ORIENTED_EDGE('',*,*,#14276,.T.);
#19030=ORIENTED_EDGE('',*,*,#14277,.F.);
#19031=ORIENTED_EDGE('',*,*,#14278,.F.);
#19032=ORIENTED_EDGE('',*,*,#14277,.T.);
#19033=ORIENTED_EDGE('',*,*,#14279,.T.);
#19034=ORIENTED_EDGE('',*,*,#14280,.F.);
#19035=ORIENTED_EDGE('',*,*,#14281,.F.);
#19036=ORIENTED_EDGE('',*,*,#14280,.T.);
#19037=ORIENTED_EDGE('',*,*,#14282,.T.);
#19038=ORIENTED_EDGE('',*,*,#14272,.F.);
#19039=ORIENTED_EDGE('',*,*,#14282,.F.);
#19040=ORIENTED_EDGE('',*,*,#14279,.F.);
#19041=ORIENTED_EDGE('',*,*,#14276,.F.);
#19042=ORIENTED_EDGE('',*,*,#14273,.F.);
#19043=ORIENTED_EDGE('',*,*,#14283,.F.);
#19044=ORIENTED_EDGE('',*,*,#14284,.T.);
#19045=ORIENTED_EDGE('',*,*,#14285,.T.);
#19046=ORIENTED_EDGE('',*,*,#14286,.F.);
#19047=ORIENTED_EDGE('',*,*,#14287,.F.);
#19048=ORIENTED_EDGE('',*,*,#14286,.T.);
#19049=ORIENTED_EDGE('',*,*,#14288,.T.);
#19050=ORIENTED_EDGE('',*,*,#14289,.F.);
#19051=ORIENTED_EDGE('',*,*,#14290,.F.);
#19052=ORIENTED_EDGE('',*,*,#14289,.T.);
#19053=ORIENTED_EDGE('',*,*,#14291,.T.);
#19054=ORIENTED_EDGE('',*,*,#14292,.F.);
#19055=ORIENTED_EDGE('',*,*,#14293,.F.);
#19056=ORIENTED_EDGE('',*,*,#14292,.T.);
#19057=ORIENTED_EDGE('',*,*,#14294,.T.);
#19058=ORIENTED_EDGE('',*,*,#14284,.F.);
#19059=ORIENTED_EDGE('',*,*,#14294,.F.);
#19060=ORIENTED_EDGE('',*,*,#14291,.F.);
#19061=ORIENTED_EDGE('',*,*,#14288,.F.);
#19062=ORIENTED_EDGE('',*,*,#14285,.F.);
#19063=ORIENTED_EDGE('',*,*,#14295,.F.);
#19064=ORIENTED_EDGE('',*,*,#14296,.T.);
#19065=ORIENTED_EDGE('',*,*,#14297,.T.);
#19066=ORIENTED_EDGE('',*,*,#14298,.F.);
#19067=ORIENTED_EDGE('',*,*,#14299,.F.);
#19068=ORIENTED_EDGE('',*,*,#14298,.T.);
#19069=ORIENTED_EDGE('',*,*,#14300,.T.);
#19070=ORIENTED_EDGE('',*,*,#14301,.F.);
#19071=ORIENTED_EDGE('',*,*,#14302,.F.);
#19072=ORIENTED_EDGE('',*,*,#14301,.T.);
#19073=ORIENTED_EDGE('',*,*,#14303,.T.);
#19074=ORIENTED_EDGE('',*,*,#14304,.F.);
#19075=ORIENTED_EDGE('',*,*,#14305,.F.);
#19076=ORIENTED_EDGE('',*,*,#14304,.T.);
#19077=ORIENTED_EDGE('',*,*,#14306,.T.);
#19078=ORIENTED_EDGE('',*,*,#14296,.F.);
#19079=ORIENTED_EDGE('',*,*,#14306,.F.);
#19080=ORIENTED_EDGE('',*,*,#14303,.F.);
#19081=ORIENTED_EDGE('',*,*,#14300,.F.);
#19082=ORIENTED_EDGE('',*,*,#14297,.F.);
#19083=ORIENTED_EDGE('',*,*,#14307,.F.);
#19084=ORIENTED_EDGE('',*,*,#14308,.F.);
#19085=ORIENTED_EDGE('',*,*,#14309,.T.);
#19086=ORIENTED_EDGE('',*,*,#14310,.T.);
#19087=ORIENTED_EDGE('',*,*,#14311,.F.);
#19088=ORIENTED_EDGE('',*,*,#14310,.F.);
#19089=ORIENTED_EDGE('',*,*,#14312,.T.);
#19090=ORIENTED_EDGE('',*,*,#14313,.T.);
#19091=ORIENTED_EDGE('',*,*,#14314,.F.);
#19092=ORIENTED_EDGE('',*,*,#14313,.F.);
#19093=ORIENTED_EDGE('',*,*,#14315,.T.);
#19094=ORIENTED_EDGE('',*,*,#14316,.T.);
#19095=ORIENTED_EDGE('',*,*,#14317,.F.);
#19096=ORIENTED_EDGE('',*,*,#14316,.F.);
#19097=ORIENTED_EDGE('',*,*,#14318,.T.);
#19098=ORIENTED_EDGE('',*,*,#14308,.T.);
#19099=ORIENTED_EDGE('',*,*,#14312,.F.);
#19100=ORIENTED_EDGE('',*,*,#14309,.F.);
#19101=ORIENTED_EDGE('',*,*,#14318,.F.);
#19102=ORIENTED_EDGE('',*,*,#14315,.F.);
#19103=ORIENTED_EDGE('',*,*,#14319,.T.);
#19104=ORIENTED_EDGE('',*,*,#14320,.T.);
#19105=ORIENTED_EDGE('',*,*,#14321,.F.);
#19106=ORIENTED_EDGE('',*,*,#14320,.F.);
#19107=ORIENTED_EDGE('',*,*,#14322,.F.);
#19108=ORIENTED_EDGE('',*,*,#14321,.T.);
#19109=ORIENTED_EDGE('',*,*,#14323,.F.);
#19110=ORIENTED_EDGE('',*,*,#14324,.T.);
#19111=ORIENTED_EDGE('',*,*,#14322,.T.);
#19112=ORIENTED_EDGE('',*,*,#14324,.F.);
#19113=ORIENTED_EDGE('',*,*,#14053,.F.);
#19114=ORIENTED_EDGE('',*,*,#14325,.T.);
#19115=ORIENTED_EDGE('',*,*,#14323,.T.);
#19116=ORIENTED_EDGE('',*,*,#14325,.F.);
#19117=ORIENTED_EDGE('',*,*,#14062,.T.);
#19118=ORIENTED_EDGE('',*,*,#14065,.T.);
#19119=ORIENTED_EDGE('',*,*,#14055,.T.);
#19120=ORIENTED_EDGE('',*,*,#14059,.T.);
#19121=ORIENTED_EDGE('',*,*,#14074,.T.);
#19122=ORIENTED_EDGE('',*,*,#14077,.T.);
#19123=ORIENTED_EDGE('',*,*,#14067,.T.);
#19124=ORIENTED_EDGE('',*,*,#14071,.T.);
#19125=ORIENTED_EDGE('',*,*,#14086,.T.);
#19126=ORIENTED_EDGE('',*,*,#14089,.T.);
#19127=ORIENTED_EDGE('',*,*,#14079,.T.);
#19128=ORIENTED_EDGE('',*,*,#14083,.T.);
#19129=ORIENTED_EDGE('',*,*,#14098,.T.);
#19130=ORIENTED_EDGE('',*,*,#14101,.T.);
#19131=ORIENTED_EDGE('',*,*,#14091,.T.);
#19132=ORIENTED_EDGE('',*,*,#14095,.T.);
#19133=ORIENTED_EDGE('',*,*,#14110,.T.);
#19134=ORIENTED_EDGE('',*,*,#14113,.T.);
#19135=ORIENTED_EDGE('',*,*,#14103,.T.);
#19136=ORIENTED_EDGE('',*,*,#14107,.T.);
#19137=ORIENTED_EDGE('',*,*,#14122,.T.);
#19138=ORIENTED_EDGE('',*,*,#14125,.T.);
#19139=ORIENTED_EDGE('',*,*,#14115,.T.);
#19140=ORIENTED_EDGE('',*,*,#14119,.T.);
#19141=ORIENTED_EDGE('',*,*,#14134,.T.);
#19142=ORIENTED_EDGE('',*,*,#14137,.T.);
#19143=ORIENTED_EDGE('',*,*,#14127,.T.);
#19144=ORIENTED_EDGE('',*,*,#14131,.T.);
#19145=ORIENTED_EDGE('',*,*,#14146,.T.);
#19146=ORIENTED_EDGE('',*,*,#14149,.T.);
#19147=ORIENTED_EDGE('',*,*,#14139,.T.);
#19148=ORIENTED_EDGE('',*,*,#14143,.T.);
#19149=ORIENTED_EDGE('',*,*,#14158,.T.);
#19150=ORIENTED_EDGE('',*,*,#14161,.T.);
#19151=ORIENTED_EDGE('',*,*,#14151,.T.);
#19152=ORIENTED_EDGE('',*,*,#14155,.T.);
#19153=ORIENTED_EDGE('',*,*,#14170,.T.);
#19154=ORIENTED_EDGE('',*,*,#14173,.T.);
#19155=ORIENTED_EDGE('',*,*,#14163,.T.);
#19156=ORIENTED_EDGE('',*,*,#14167,.T.);
#19157=ORIENTED_EDGE('',*,*,#14182,.T.);
#19158=ORIENTED_EDGE('',*,*,#14185,.T.);
#19159=ORIENTED_EDGE('',*,*,#14175,.T.);
#19160=ORIENTED_EDGE('',*,*,#14179,.T.);
#19161=ORIENTED_EDGE('',*,*,#14194,.T.);
#19162=ORIENTED_EDGE('',*,*,#14197,.T.);
#19163=ORIENTED_EDGE('',*,*,#14187,.T.);
#19164=ORIENTED_EDGE('',*,*,#14191,.T.);
#19165=ORIENTED_EDGE('',*,*,#14206,.T.);
#19166=ORIENTED_EDGE('',*,*,#14209,.T.);
#19167=ORIENTED_EDGE('',*,*,#14199,.T.);
#19168=ORIENTED_EDGE('',*,*,#14203,.T.);
#19169=ORIENTED_EDGE('',*,*,#14218,.T.);
#19170=ORIENTED_EDGE('',*,*,#14221,.T.);
#19171=ORIENTED_EDGE('',*,*,#14211,.T.);
#19172=ORIENTED_EDGE('',*,*,#14215,.T.);
#19173=ORIENTED_EDGE('',*,*,#14230,.T.);
#19174=ORIENTED_EDGE('',*,*,#14233,.T.);
#19175=ORIENTED_EDGE('',*,*,#14223,.T.);
#19176=ORIENTED_EDGE('',*,*,#14227,.T.);
#19177=ORIENTED_EDGE('',*,*,#14242,.T.);
#19178=ORIENTED_EDGE('',*,*,#14245,.T.);
#19179=ORIENTED_EDGE('',*,*,#14235,.T.);
#19180=ORIENTED_EDGE('',*,*,#14239,.T.);
#19181=ORIENTED_EDGE('',*,*,#14254,.T.);
#19182=ORIENTED_EDGE('',*,*,#14257,.T.);
#19183=ORIENTED_EDGE('',*,*,#14247,.T.);
#19184=ORIENTED_EDGE('',*,*,#14251,.T.);
#19185=ORIENTED_EDGE('',*,*,#14266,.T.);
#19186=ORIENTED_EDGE('',*,*,#14269,.T.);
#19187=ORIENTED_EDGE('',*,*,#14259,.T.);
#19188=ORIENTED_EDGE('',*,*,#14263,.T.);
#19189=ORIENTED_EDGE('',*,*,#14278,.T.);
#19190=ORIENTED_EDGE('',*,*,#14281,.T.);
#19191=ORIENTED_EDGE('',*,*,#14271,.T.);
#19192=ORIENTED_EDGE('',*,*,#14275,.T.);
#19193=ORIENTED_EDGE('',*,*,#14290,.T.);
#19194=ORIENTED_EDGE('',*,*,#14293,.T.);
#19195=ORIENTED_EDGE('',*,*,#14283,.T.);
#19196=ORIENTED_EDGE('',*,*,#14287,.T.);
#19197=ORIENTED_EDGE('',*,*,#14302,.T.);
#19198=ORIENTED_EDGE('',*,*,#14305,.T.);
#19199=ORIENTED_EDGE('',*,*,#14295,.T.);
#19200=ORIENTED_EDGE('',*,*,#14299,.T.);
#19201=ORIENTED_EDGE('',*,*,#14314,.T.);
#19202=ORIENTED_EDGE('',*,*,#14317,.T.);
#19203=ORIENTED_EDGE('',*,*,#14307,.T.);
#19204=ORIENTED_EDGE('',*,*,#14311,.T.);
#19205=ORIENTED_EDGE('',*,*,#14054,.T.);
#19206=ORIENTED_EDGE('',*,*,#14326,.T.);
#19207=ORIENTED_EDGE('',*,*,#14327,.F.);
#19208=ORIENTED_EDGE('',*,*,#14326,.F.);
#19209=ORIENTED_EDGE('',*,*,#14327,.T.);
#19210=ORIENTED_EDGE('',*,*,#14328,.T.);
#19211=ORIENTED_EDGE('',*,*,#14329,.F.);
#19212=ORIENTED_EDGE('',*,*,#14328,.F.);
#19213=ORIENTED_EDGE('',*,*,#14329,.T.);
#19214=ORIENTED_EDGE('',*,*,#14330,.F.);
#19215=ORIENTED_EDGE('',*,*,#14330,.T.);
#19216=ORIENTED_EDGE('',*,*,#14331,.T.);
#19217=ORIENTED_EDGE('',*,*,#14332,.F.);
#19218=ORIENTED_EDGE('',*,*,#14331,.F.);
#19219=ORIENTED_EDGE('',*,*,#14319,.F.);
#19220=ORIENTED_EDGE('',*,*,#14332,.T.);
#25008=CONICAL_SURFACE('',#27396,3.08422464300993,0.974356912318788);
#25009=CONICAL_SURFACE('',#27400,3.2985,0.377917497842688);
#25010=CONICAL_SURFACE('',#27563,3.447,0.785398163397451);
#25011=CONICAL_SURFACE('',#27566,1.6023112,0.798216012485968);
#25012=CONICAL_SURFACE('',#27568,1.4090882,0.0259641639514023);
#25421=ADVANCED_FACE('',(#2833),#25008,.T.);
#25422=ADVANCED_FACE('',(#2834),#25009,.T.);
#25423=ADVANCED_FACE('',(#2835,#1580),#1804,.T.);
#25424=ADVANCED_FACE('',(#2836),#1805,.F.);
#25425=ADVANCED_FACE('',(#2837),#1806,.F.);
#25426=ADVANCED_FACE('',(#2838),#1807,.F.);
#25427=ADVANCED_FACE('',(#2839),#1808,.F.);
#25428=ADVANCED_FACE('',(#2840),#1809,.F.);
#25429=ADVANCED_FACE('',(#2841),#1810,.F.);
#25430=ADVANCED_FACE('',(#2842),#1811,.F.);
#25431=ADVANCED_FACE('',(#2843),#1812,.F.);
#25432=ADVANCED_FACE('',(#2844),#1813,.F.);
#25433=ADVANCED_FACE('',(#2845),#1814,.F.);
#25434=ADVANCED_FACE('',(#2846),#1815,.F.);
#25435=ADVANCED_FACE('',(#2847),#1816,.F.);
#25436=ADVANCED_FACE('',(#2848),#1817,.F.);
#25437=ADVANCED_FACE('',(#2849),#1818,.F.);
#25438=ADVANCED_FACE('',(#2850),#1819,.F.);
#25439=ADVANCED_FACE('',(#2851),#1820,.F.);
#25440=ADVANCED_FACE('',(#2852),#1821,.F.);
#25441=ADVANCED_FACE('',(#2853),#1822,.F.);
#25442=ADVANCED_FACE('',(#2854),#1823,.F.);
#25443=ADVANCED_FACE('',(#2855),#1824,.F.);
#25444=ADVANCED_FACE('',(#2856),#1825,.F.);
#25445=ADVANCED_FACE('',(#2857),#1826,.F.);
#25446=ADVANCED_FACE('',(#2858),#1827,.F.);
#25447=ADVANCED_FACE('',(#2859),#1828,.F.);
#25448=ADVANCED_FACE('',(#2860),#1829,.F.);
#25449=ADVANCED_FACE('',(#2861),#1830,.F.);
#25450=ADVANCED_FACE('',(#2862),#1831,.F.);
#25451=ADVANCED_FACE('',(#2863),#1832,.F.);
#25452=ADVANCED_FACE('',(#2864),#1833,.F.);
#25453=ADVANCED_FACE('',(#2865),#1834,.F.);
#25454=ADVANCED_FACE('',(#2866),#1835,.F.);
#25455=ADVANCED_FACE('',(#2867),#1836,.F.);
#25456=ADVANCED_FACE('',(#2868),#1837,.F.);
#25457=ADVANCED_FACE('',(#2869),#1838,.F.);
#25458=ADVANCED_FACE('',(#2870),#1839,.F.);
#25459=ADVANCED_FACE('',(#2871),#1840,.F.);
#25460=ADVANCED_FACE('',(#2872),#1841,.F.);
#25461=ADVANCED_FACE('',(#2873),#1842,.F.);
#25462=ADVANCED_FACE('',(#2874),#1843,.F.);
#25463=ADVANCED_FACE('',(#2875),#1844,.F.);
#25464=ADVANCED_FACE('',(#2876),#1845,.F.);
#25465=ADVANCED_FACE('',(#2877),#1846,.F.);
#25466=ADVANCED_FACE('',(#2878),#1847,.F.);
#25467=ADVANCED_FACE('',(#2879),#1848,.F.);
#25468=ADVANCED_FACE('',(#2880),#1849,.F.);
#25469=ADVANCED_FACE('',(#2881),#1850,.F.);
#25470=ADVANCED_FACE('',(#2882),#1851,.F.);
#25471=ADVANCED_FACE('',(#2883),#1852,.F.);
#25472=ADVANCED_FACE('',(#2884),#1853,.F.);
#25473=ADVANCED_FACE('',(#2885),#1854,.F.);
#25474=ADVANCED_FACE('',(#2886),#1855,.F.);
#25475=ADVANCED_FACE('',(#2887),#1856,.F.);
#25476=ADVANCED_FACE('',(#2888),#1857,.F.);
#25477=ADVANCED_FACE('',(#2889),#1858,.F.);
#25478=ADVANCED_FACE('',(#2890),#1859,.F.);
#25479=ADVANCED_FACE('',(#2891),#1860,.F.);
#25480=ADVANCED_FACE('',(#2892),#1861,.F.);
#25481=ADVANCED_FACE('',(#2893),#1862,.F.);
#25482=ADVANCED_FACE('',(#2894),#1863,.F.);
#25483=ADVANCED_FACE('',(#2895),#1864,.F.);
#25484=ADVANCED_FACE('',(#2896),#1865,.F.);
#25485=ADVANCED_FACE('',(#2897),#1866,.F.);
#25486=ADVANCED_FACE('',(#2898),#1867,.F.);
#25487=ADVANCED_FACE('',(#2899),#1868,.F.);
#25488=ADVANCED_FACE('',(#2900),#1869,.F.);
#25489=ADVANCED_FACE('',(#2901),#1870,.F.);
#25490=ADVANCED_FACE('',(#2902),#1871,.F.);
#25491=ADVANCED_FACE('',(#2903),#1872,.F.);
#25492=ADVANCED_FACE('',(#2904),#1873,.F.);
#25493=ADVANCED_FACE('',(#2905),#1874,.F.);
#25494=ADVANCED_FACE('',(#2906),#1875,.F.);
#25495=ADVANCED_FACE('',(#2907),#1876,.F.);
#25496=ADVANCED_FACE('',(#2908),#1877,.F.);
#25497=ADVANCED_FACE('',(#2909),#1878,.F.);
#25498=ADVANCED_FACE('',(#2910),#1879,.F.);
#25499=ADVANCED_FACE('',(#2911),#1880,.F.);
#25500=ADVANCED_FACE('',(#2912),#1881,.F.);
#25501=ADVANCED_FACE('',(#2913),#1882,.F.);
#25502=ADVANCED_FACE('',(#2914),#1883,.F.);
#25503=ADVANCED_FACE('',(#2915),#1884,.F.);
#25504=ADVANCED_FACE('',(#2916),#1885,.F.);
#25505=ADVANCED_FACE('',(#2917),#1886,.F.);
#25506=ADVANCED_FACE('',(#2918),#1887,.F.);
#25507=ADVANCED_FACE('',(#2919),#1888,.F.);
#25508=ADVANCED_FACE('',(#2920),#1889,.F.);
#25509=ADVANCED_FACE('',(#2921),#1890,.F.);
#25510=ADVANCED_FACE('',(#2922),#1891,.F.);
#25511=ADVANCED_FACE('',(#2923),#1892,.F.);
#25512=ADVANCED_FACE('',(#2924),#1893,.F.);
#25513=ADVANCED_FACE('',(#2925),#1894,.F.);
#25514=ADVANCED_FACE('',(#2926),#1895,.F.);
#25515=ADVANCED_FACE('',(#2927),#1896,.F.);
#25516=ADVANCED_FACE('',(#2928),#1897,.F.);
#25517=ADVANCED_FACE('',(#2929),#1898,.F.);
#25518=ADVANCED_FACE('',(#2930),#1899,.F.);
#25519=ADVANCED_FACE('',(#2931),#1900,.F.);
#25520=ADVANCED_FACE('',(#2932),#1901,.F.);
#25521=ADVANCED_FACE('',(#2933),#1902,.F.);
#25522=ADVANCED_FACE('',(#2934),#1903,.F.);
#25523=ADVANCED_FACE('',(#2935),#1904,.F.);
#25524=ADVANCED_FACE('',(#2936),#1905,.F.);
#25525=ADVANCED_FACE('',(#2937),#1906,.F.);
#25526=ADVANCED_FACE('',(#2938),#1907,.F.);
#25527=ADVANCED_FACE('',(#2939),#1908,.F.);
#25528=ADVANCED_FACE('',(#2940),#1909,.F.);
#25529=ADVANCED_FACE('',(#2941),#1910,.F.);
#25530=ADVANCED_FACE('',(#2942),#1155,.F.);
#25531=ADVANCED_FACE('',(#2943),#1911,.F.);
#25532=ADVANCED_FACE('',(#2944),#1156,.F.);
#25533=ADVANCED_FACE('',(#2945),#1912,.F.);
#25534=ADVANCED_FACE('',(#2946),#1157,.F.);
#25535=ADVANCED_FACE('',(#2947,#1581),#1913,.T.);
#25536=ADVANCED_FACE('',(#2948),#25010,.T.);
#25537=ADVANCED_FACE('',(#2949,#1582,#1583,#1584,#1585,#1586,#1587,#1588,
#1589,#1590,#1591,#1592,#1593,#1594,#1595,#1596,#1597,#1598,#1599,#1600,
#1601,#1602,#1603),#1158,.T.);
#25538=ADVANCED_FACE('',(#2950),#25011,.F.);
#25539=ADVANCED_FACE('',(#2951),#25012,.F.);
#25540=ADVANCED_FACE('',(#2952,#1604),#1914,.T.);
#25541=ADVANCED_FACE('',(#2953),#1159,.F.);
#25542=ADVANCED_FACE('',(#2954,#1605),#1915,.T.);
#26666=CLOSED_SHELL('',(#25421,#25422,#25423,#25424,#25425,#25426,#25427,
#25428,#25429,#25430,#25431,#25432,#25433,#25434,#25435,#25436,#25437,#25438,
#25439,#25440,#25441,#25442,#25443,#25444,#25445,#25446,#25447,#25448,#25449,
#25450,#25451,#25452,#25453,#25454,#25455,#25456,#25457,#25458,#25459,#25460,
#25461,#25462,#25463,#25464,#25465,#25466,#25467,#25468,#25469,#25470,#25471,
#25472,#25473,#25474,#25475,#25476,#25477,#25478,#25479,#25480,#25481,#25482,
#25483,#25484,#25485,#25486,#25487,#25488,#25489,#25490,#25491,#25492,#25493,
#25494,#25495,#25496,#25497,#25498,#25499,#25500,#25501,#25502,#25503,#25504,
#25505,#25506,#25507,#25508,#25509,#25510,#25511,#25512,#25513,#25514,#25515,
#25516,#25517,#25518,#25519,#25520,#25521,#25522,#25523,#25524,#25525,#25526,
#25527,#25528,#25529,#25530,#25531,#25532,#25533,#25534,#25535,#25536,#25537,
#25538,#25539,#25540,#25541,#25542));
#27395=AXIS2_PLACEMENT_3D('',#39436,#30797,#30798);
#27396=AXIS2_PLACEMENT_3D('',#39437,#30799,#30800);
#27397=AXIS2_PLACEMENT_3D('',#39439,#30801,#30802);
#27398=AXIS2_PLACEMENT_3D('',#39443,#30804,#30805);
#27399=AXIS2_PLACEMENT_3D('',#39444,#30806,#30807);
#27400=AXIS2_PLACEMENT_3D('',#39445,#30808,#30809);
#27401=AXIS2_PLACEMENT_3D('',#39448,#30811,#30812);
#27402=AXIS2_PLACEMENT_3D('',#39449,#30813,#30814);
#27403=AXIS2_PLACEMENT_3D('',#39451,#30815,#30816);
#27404=AXIS2_PLACEMENT_3D('',#39452,#30817,#30818);
#27405=AXIS2_PLACEMENT_3D('',#39461,#30823,#30824);
#27406=AXIS2_PLACEMENT_3D('',#39463,#30825,#30826);
#27407=AXIS2_PLACEMENT_3D('',#39467,#30829,#30830);
#27408=AXIS2_PLACEMENT_3D('',#39473,#30834,#30835);
#27409=AXIS2_PLACEMENT_3D('',#39474,#30836,#30837);
#27410=AXIS2_PLACEMENT_3D('',#39476,#30839,#30840);
#27411=AXIS2_PLACEMENT_3D('',#39477,#30841,#30842);
#27412=AXIS2_PLACEMENT_3D('',#39486,#30847,#30848);
#27413=AXIS2_PLACEMENT_3D('',#39488,#30849,#30850);
#27414=AXIS2_PLACEMENT_3D('',#39492,#30853,#30854);
#27415=AXIS2_PLACEMENT_3D('',#39498,#30858,#30859);
#27416=AXIS2_PLACEMENT_3D('',#39499,#30860,#30861);
#27417=AXIS2_PLACEMENT_3D('',#39501,#30863,#30864);
#27418=AXIS2_PLACEMENT_3D('',#39502,#30865,#30866);
#27419=AXIS2_PLACEMENT_3D('',#39511,#30871,#30872);
#27420=AXIS2_PLACEMENT_3D('',#39513,#30873,#30874);
#27421=AXIS2_PLACEMENT_3D('',#39517,#30877,#30878);
#27422=AXIS2_PLACEMENT_3D('',#39523,#30882,#30883);
#27423=AXIS2_PLACEMENT_3D('',#39524,#30884,#30885);
#27424=AXIS2_PLACEMENT_3D('',#39526,#30887,#30888);
#27425=AXIS2_PLACEMENT_3D('',#39527,#30889,#30890);
#27426=AXIS2_PLACEMENT_3D('',#39536,#30895,#30896);
#27427=AXIS2_PLACEMENT_3D('',#39538,#30897,#30898);
#27428=AXIS2_PLACEMENT_3D('',#39542,#30901,#30902);
#27429=AXIS2_PLACEMENT_3D('',#39548,#30906,#30907);
#27430=AXIS2_PLACEMENT_3D('',#39549,#30908,#30909);
#27431=AXIS2_PLACEMENT_3D('',#39551,#30911,#30912);
#27432=AXIS2_PLACEMENT_3D('',#39552,#30913,#30914);
#27433=AXIS2_PLACEMENT_3D('',#39561,#30919,#30920);
#27434=AXIS2_PLACEMENT_3D('',#39563,#30921,#30922);
#27435=AXIS2_PLACEMENT_3D('',#39567,#30925,#30926);
#27436=AXIS2_PLACEMENT_3D('',#39573,#30930,#30931);
#27437=AXIS2_PLACEMENT_3D('',#39574,#30932,#30933);
#27438=AXIS2_PLACEMENT_3D('',#39576,#30935,#30936);
#27439=AXIS2_PLACEMENT_3D('',#39577,#30937,#30938);
#27440=AXIS2_PLACEMENT_3D('',#39586,#30943,#30944);
#27441=AXIS2_PLACEMENT_3D('',#39588,#30945,#30946);
#27442=AXIS2_PLACEMENT_3D('',#39592,#30949,#30950);
#27443=AXIS2_PLACEMENT_3D('',#39598,#30954,#30955);
#27444=AXIS2_PLACEMENT_3D('',#39599,#30956,#30957);
#27445=AXIS2_PLACEMENT_3D('',#39601,#30959,#30960);
#27446=AXIS2_PLACEMENT_3D('',#39602,#30961,#30962);
#27447=AXIS2_PLACEMENT_3D('',#39611,#30967,#30968);
#27448=AXIS2_PLACEMENT_3D('',#39613,#30969,#30970);
#27449=AXIS2_PLACEMENT_3D('',#39617,#30973,#30974);
#27450=AXIS2_PLACEMENT_3D('',#39623,#30978,#30979);
#27451=AXIS2_PLACEMENT_3D('',#39624,#30980,#30981);
#27452=AXIS2_PLACEMENT_3D('',#39626,#30983,#30984);
#27453=AXIS2_PLACEMENT_3D('',#39627,#30985,#30986);
#27454=AXIS2_PLACEMENT_3D('',#39636,#30991,#30992);
#27455=AXIS2_PLACEMENT_3D('',#39638,#30993,#30994);
#27456=AXIS2_PLACEMENT_3D('',#39642,#30997,#30998);
#27457=AXIS2_PLACEMENT_3D('',#39648,#31002,#31003);
#27458=AXIS2_PLACEMENT_3D('',#39649,#31004,#31005);
#27459=AXIS2_PLACEMENT_3D('',#39651,#31007,#31008);
#27460=AXIS2_PLACEMENT_3D('',#39652,#31009,#31010);
#27461=AXIS2_PLACEMENT_3D('',#39661,#31015,#31016);
#27462=AXIS2_PLACEMENT_3D('',#39663,#31017,#31018);
#27463=AXIS2_PLACEMENT_3D('',#39667,#31021,#31022);
#27464=AXIS2_PLACEMENT_3D('',#39673,#31026,#31027);
#27465=AXIS2_PLACEMENT_3D('',#39674,#31028,#31029);
#27466=AXIS2_PLACEMENT_3D('',#39676,#31031,#31032);
#27467=AXIS2_PLACEMENT_3D('',#39677,#31033,#31034);
#27468=AXIS2_PLACEMENT_3D('',#39686,#31039,#31040);
#27469=AXIS2_PLACEMENT_3D('',#39688,#31041,#31042);
#27470=AXIS2_PLACEMENT_3D('',#39692,#31045,#31046);
#27471=AXIS2_PLACEMENT_3D('',#39698,#31050,#31051);
#27472=AXIS2_PLACEMENT_3D('',#39699,#31052,#31053);
#27473=AXIS2_PLACEMENT_3D('',#39701,#31055,#31056);
#27474=AXIS2_PLACEMENT_3D('',#39702,#31057,#31058);
#27475=AXIS2_PLACEMENT_3D('',#39711,#31063,#31064);
#27476=AXIS2_PLACEMENT_3D('',#39713,#31065,#31066);
#27477=AXIS2_PLACEMENT_3D('',#39717,#31069,#31070);
#27478=AXIS2_PLACEMENT_3D('',#39723,#31074,#31075);
#27479=AXIS2_PLACEMENT_3D('',#39724,#31076,#31077);
#27480=AXIS2_PLACEMENT_3D('',#39726,#31079,#31080);
#27481=AXIS2_PLACEMENT_3D('',#39727,#31081,#31082);
#27482=AXIS2_PLACEMENT_3D('',#39736,#31087,#31088);
#27483=AXIS2_PLACEMENT_3D('',#39738,#31089,#31090);
#27484=AXIS2_PLACEMENT_3D('',#39742,#31093,#31094);
#27485=AXIS2_PLACEMENT_3D('',#39748,#31098,#31099);
#27486=AXIS2_PLACEMENT_3D('',#39749,#31100,#31101);
#27487=AXIS2_PLACEMENT_3D('',#39751,#31103,#31104);
#27488=AXIS2_PLACEMENT_3D('',#39752,#31105,#31106);
#27489=AXIS2_PLACEMENT_3D('',#39761,#31111,#31112);
#27490=AXIS2_PLACEMENT_3D('',#39763,#31113,#31114);
#27491=AXIS2_PLACEMENT_3D('',#39767,#31117,#31118);
#27492=AXIS2_PLACEMENT_3D('',#39773,#31122,#31123);
#27493=AXIS2_PLACEMENT_3D('',#39774,#31124,#31125);
#27494=AXIS2_PLACEMENT_3D('',#39776,#31127,#31128);
#27495=AXIS2_PLACEMENT_3D('',#39777,#31129,#31130);
#27496=AXIS2_PLACEMENT_3D('',#39786,#31135,#31136);
#27497=AXIS2_PLACEMENT_3D('',#39788,#31137,#31138);
#27498=AXIS2_PLACEMENT_3D('',#39792,#31141,#31142);
#27499=AXIS2_PLACEMENT_3D('',#39798,#31146,#31147);
#27500=AXIS2_PLACEMENT_3D('',#39799,#31148,#31149);
#27501=AXIS2_PLACEMENT_3D('',#39801,#31151,#31152);
#27502=AXIS2_PLACEMENT_3D('',#39802,#31153,#31154);
#27503=AXIS2_PLACEMENT_3D('',#39811,#31159,#31160);
#27504=AXIS2_PLACEMENT_3D('',#39813,#31161,#31162);
#27505=AXIS2_PLACEMENT_3D('',#39817,#31165,#31166);
#27506=AXIS2_PLACEMENT_3D('',#39823,#31170,#31171);
#27507=AXIS2_PLACEMENT_3D('',#39824,#31172,#31173);
#27508=AXIS2_PLACEMENT_3D('',#39826,#31175,#31176);
#27509=AXIS2_PLACEMENT_3D('',#39827,#31177,#31178);
#27510=AXIS2_PLACEMENT_3D('',#39836,#31183,#31184);
#27511=AXIS2_PLACEMENT_3D('',#39838,#31185,#31186);
#27512=AXIS2_PLACEMENT_3D('',#39842,#31189,#31190);
#27513=AXIS2_PLACEMENT_3D('',#39848,#31194,#31195);
#27514=AXIS2_PLACEMENT_3D('',#39849,#31196,#31197);
#27515=AXIS2_PLACEMENT_3D('',#39851,#31199,#31200);
#27516=AXIS2_PLACEMENT_3D('',#39852,#31201,#31202);
#27517=AXIS2_PLACEMENT_3D('',#39861,#31207,#31208);
#27518=AXIS2_PLACEMENT_3D('',#39863,#31209,#31210);
#27519=AXIS2_PLACEMENT_3D('',#39867,#31213,#31214);
#27520=AXIS2_PLACEMENT_3D('',#39873,#31218,#31219);
#27521=AXIS2_PLACEMENT_3D('',#39874,#31220,#31221);
#27522=AXIS2_PLACEMENT_3D('',#39876,#31223,#31224);
#27523=AXIS2_PLACEMENT_3D('',#39877,#31225,#31226);
#27524=AXIS2_PLACEMENT_3D('',#39886,#31231,#31232);
#27525=AXIS2_PLACEMENT_3D('',#39888,#31233,#31234);
#27526=AXIS2_PLACEMENT_3D('',#39892,#31237,#31238);
#27527=AXIS2_PLACEMENT_3D('',#39898,#31242,#31243);
#27528=AXIS2_PLACEMENT_3D('',#39899,#31244,#31245);
#27529=AXIS2_PLACEMENT_3D('',#39901,#31247,#31248);
#27530=AXIS2_PLACEMENT_3D('',#39902,#31249,#31250);
#27531=AXIS2_PLACEMENT_3D('',#39911,#31255,#31256);
#27532=AXIS2_PLACEMENT_3D('',#39913,#31257,#31258);
#27533=AXIS2_PLACEMENT_3D('',#39917,#31261,#31262);
#27534=AXIS2_PLACEMENT_3D('',#39923,#31266,#31267);
#27535=AXIS2_PLACEMENT_3D('',#39924,#31268,#31269);
#27536=AXIS2_PLACEMENT_3D('',#39926,#31271,#31272);
#27537=AXIS2_PLACEMENT_3D('',#39927,#31273,#31274);
#27538=AXIS2_PLACEMENT_3D('',#39936,#31279,#31280);
#27539=AXIS2_PLACEMENT_3D('',#39938,#31281,#31282);
#27540=AXIS2_PLACEMENT_3D('',#39942,#31285,#31286);
#27541=AXIS2_PLACEMENT_3D('',#39948,#31290,#31291);
#27542=AXIS2_PLACEMENT_3D('',#39949,#31292,#31293);
#27543=AXIS2_PLACEMENT_3D('',#39951,#31295,#31296);
#27544=AXIS2_PLACEMENT_3D('',#39952,#31297,#31298);
#27545=AXIS2_PLACEMENT_3D('',#39961,#31303,#31304);
#27546=AXIS2_PLACEMENT_3D('',#39963,#31305,#31306);
#27547=AXIS2_PLACEMENT_3D('',#39967,#31309,#31310);
#27548=AXIS2_PLACEMENT_3D('',#39973,#31314,#31315);
#27549=AXIS2_PLACEMENT_3D('',#39974,#31316,#31317);
#27550=AXIS2_PLACEMENT_3D('',#39976,#31319,#31320);
#27551=AXIS2_PLACEMENT_3D('',#39977,#31321,#31322);
#27552=AXIS2_PLACEMENT_3D('',#39986,#31327,#31328);
#27553=AXIS2_PLACEMENT_3D('',#40007,#31329,#31330);
#27554=AXIS2_PLACEMENT_3D('',#40009,#31332,#31333);
#27555=AXIS2_PLACEMENT_3D('',#40015,#31337,#31338);
#27556=AXIS2_PLACEMENT_3D('',#40034,#31339,#31340);
#27557=AXIS2_PLACEMENT_3D('',#40035,#31341,#31342);
#27558=AXIS2_PLACEMENT_3D('',#40036,#31343,#31344);
#27559=AXIS2_PLACEMENT_3D('',#40038,#31345,#31346);
#27560=AXIS2_PLACEMENT_3D('',#40041,#31348,#31349);
#27561=AXIS2_PLACEMENT_3D('',#40042,#31350,#31351);
#27562=AXIS2_PLACEMENT_3D('',#40044,#31352,#31353);
#27563=AXIS2_PLACEMENT_3D('',#40045,#31354,#31355);
#27564=AXIS2_PLACEMENT_3D('',#40047,#31356,#31357);
#27565=AXIS2_PLACEMENT_3D('',#40049,#31359,#31360);
#27566=AXIS2_PLACEMENT_3D('',#40051,#31362,#31363);
#27567=AXIS2_PLACEMENT_3D('',#40054,#31365,#31366);
#27568=AXIS2_PLACEMENT_3D('',#40055,#31367,#31368);
#27569=AXIS2_PLACEMENT_3D('',#40058,#31370,#31371);
#27570=AXIS2_PLACEMENT_3D('',#40059,#31372,#31373);
#27571=AXIS2_PLACEMENT_3D('',#40061,#31374,#31375);
#27572=AXIS2_PLACEMENT_3D('',#40062,#31376,#31377);
#27573=AXIS2_PLACEMENT_3D('',#40065,#31379,#31380);
#27574=AXIS2_PLACEMENT_3D('',#40066,#31381,#31382);
#30797=DIRECTION('axis',(0.,0.,1.));
#30798=DIRECTION('refdir',(1.,0.,0.));
#30799=DIRECTION('center_axis',(-1.,0.,0.));
#30800=DIRECTION('ref_axis',(0.,-1.,0.));
#30801=DIRECTION('center_axis',(-1.,0.,0.));
#30802=DIRECTION('ref_axis',(0.,-1.,0.));
#30803=DIRECTION('',(-0.561700222361827,0.827340836776884,1.0132003075627E-16));
#30804=DIRECTION('center_axis',(1.,0.,0.));
#30805=DIRECTION('ref_axis',(0.,-1.,0.));
#30806=DIRECTION('center_axis',(1.,0.,0.));
#30807=DIRECTION('ref_axis',(0.,-1.,0.));
#30808=DIRECTION('center_axis',(-1.,0.,0.));
#30809=DIRECTION('ref_axis',(0.,1.,0.));
#30810=DIRECTION('',(-0.929435063973188,-0.368985720397356,-4.51877181415702E-17));
#30811=DIRECTION('center_axis',(1.,0.,0.));
#30812=DIRECTION('ref_axis',(0.,0.,-1.));
#30813=DIRECTION('center_axis',(1.,0.,0.));
#30814=DIRECTION('ref_axis',(0.,0.,-1.));
#30815=DIRECTION('center_axis',(1.,0.,0.));
#30816=DIRECTION('ref_axis',(0.,0.,-1.));
#30817=DIRECTION('center_axis',(0.,1.,0.));
#30818=DIRECTION('ref_axis',(1.,0.,0.));
#30819=DIRECTION('',(1.,0.,0.));
#30820=DIRECTION('',(0.,0.,-1.));
#30821=DIRECTION('',(1.,0.,0.));
#30822=DIRECTION('',(0.,0.,-1.));
#30823=DIRECTION('center_axis',(1.,0.,0.));
#30824=DIRECTION('ref_axis',(0.,-1.,0.));
#30825=DIRECTION('center_axis',(1.,0.,0.));
#30826=DIRECTION('ref_axis',(0.,1.,0.));
#30827=DIRECTION('',(0.,-1.,0.));
#30828=DIRECTION('',(0.,0.,-1.));
#30829=DIRECTION('center_axis',(0.,-1.,0.));
#30830=DIRECTION('ref_axis',(-1.,0.,0.));
#30831=DIRECTION('',(-1.,0.,0.));
#30832=DIRECTION('',(-1.,0.,0.));
#30833=DIRECTION('',(0.,0.,-1.));
#30834=DIRECTION('center_axis',(-1.,0.,0.));
#30835=DIRECTION('ref_axis',(0.,1.,0.));
#30836=DIRECTION('center_axis',(-1.,0.,0.));
#30837=DIRECTION('ref_axis',(0.,1.,0.));
#30838=DIRECTION('',(0.,1.,0.));
#30839=DIRECTION('center_axis',(0.,0.,-1.));
#30840=DIRECTION('ref_axis',(-1.,0.,0.));
#30841=DIRECTION('center_axis',(0.,1.,0.));
#30842=DIRECTION('ref_axis',(1.,0.,0.));
#30843=DIRECTION('',(1.,0.,0.));
#30844=DIRECTION('',(0.,0.,-1.));
#30845=DIRECTION('',(1.,0.,0.));
#30846=DIRECTION('',(0.,0.,-1.));
#30847=DIRECTION('center_axis',(1.,0.,0.));
#30848=DIRECTION('ref_axis',(0.,-1.,0.));
#30849=DIRECTION('center_axis',(1.,0.,0.));
#30850=DIRECTION('ref_axis',(0.,1.,0.));
#30851=DIRECTION('',(0.,-1.,0.));
#30852=DIRECTION('',(0.,0.,-1.));
#30853=DIRECTION('center_axis',(0.,-1.,0.));
#30854=DIRECTION('ref_axis',(-1.,0.,0.));
#30855=DIRECTION('',(-1.,0.,0.));
#30856=DIRECTION('',(-1.,0.,0.));
#30857=DIRECTION('',(0.,0.,-1.));
#30858=DIRECTION('center_axis',(-1.,0.,0.));
#30859=DIRECTION('ref_axis',(0.,1.,0.));
#30860=DIRECTION('center_axis',(-1.,0.,0.));
#30861=DIRECTION('ref_axis',(0.,1.,0.));
#30862=DIRECTION('',(0.,1.,0.));
#30863=DIRECTION('center_axis',(0.,0.,-1.));
#30864=DIRECTION('ref_axis',(-1.,0.,0.));
#30865=DIRECTION('center_axis',(0.,1.,0.));
#30866=DIRECTION('ref_axis',(1.,0.,0.));
#30867=DIRECTION('',(1.,0.,0.));
#30868=DIRECTION('',(0.,0.,-1.));
#30869=DIRECTION('',(1.,0.,0.));
#30870=DIRECTION('',(0.,0.,-1.));
#30871=DIRECTION('center_axis',(1.,0.,0.));
#30872=DIRECTION('ref_axis',(0.,-1.,0.));
#30873=DIRECTION('center_axis',(1.,0.,0.));
#30874=DIRECTION('ref_axis',(0.,1.,0.));
#30875=DIRECTION('',(0.,-1.,0.));
#30876=DIRECTION('',(0.,0.,-1.));
#30877=DIRECTION('center_axis',(0.,-1.,0.));
#30878=DIRECTION('ref_axis',(-1.,0.,0.));
#30879=DIRECTION('',(-1.,0.,0.));
#30880=DIRECTION('',(-1.,0.,0.));
#30881=DIRECTION('',(0.,0.,-1.));
#30882=DIRECTION('center_axis',(-1.,0.,0.));
#30883=DIRECTION('ref_axis',(0.,1.,0.));
#30884=DIRECTION('center_axis',(-1.,0.,0.));
#30885=DIRECTION('ref_axis',(0.,1.,0.));
#30886=DIRECTION('',(0.,1.,0.));
#30887=DIRECTION('center_axis',(0.,0.,-1.));
#30888=DIRECTION('ref_axis',(-1.,0.,0.));
#30889=DIRECTION('center_axis',(0.,1.,0.));
#30890=DIRECTION('ref_axis',(1.,0.,0.));
#30891=DIRECTION('',(1.,0.,0.));
#30892=DIRECTION('',(0.,0.,-1.));
#30893=DIRECTION('',(1.,0.,0.));
#30894=DIRECTION('',(0.,0.,-1.));
#30895=DIRECTION('center_axis',(1.,0.,0.));
#30896=DIRECTION('ref_axis',(0.,-1.,0.));
#30897=DIRECTION('center_axis',(1.,0.,0.));
#30898=DIRECTION('ref_axis',(0.,1.,0.));
#30899=DIRECTION('',(0.,-1.,0.));
#30900=DIRECTION('',(0.,0.,-1.));
#30901=DIRECTION('center_axis',(0.,-1.,0.));
#30902=DIRECTION('ref_axis',(-1.,0.,0.));
#30903=DIRECTION('',(-1.,0.,0.));
#30904=DIRECTION('',(-1.,0.,0.));
#30905=DIRECTION('',(0.,0.,-1.));
#30906=DIRECTION('center_axis',(-1.,0.,0.));
#30907=DIRECTION('ref_axis',(0.,1.,0.));
#30908=DIRECTION('center_axis',(-1.,0.,0.));
#30909=DIRECTION('ref_axis',(0.,1.,0.));
#30910=DIRECTION('',(0.,1.,0.));
#30911=DIRECTION('center_axis',(0.,0.,-1.));
#30912=DIRECTION('ref_axis',(-1.,0.,0.));
#30913=DIRECTION('center_axis',(0.,1.,0.));
#30914=DIRECTION('ref_axis',(1.,0.,0.));
#30915=DIRECTION('',(1.,0.,0.));
#30916=DIRECTION('',(0.,0.,-1.));
#30917=DIRECTION('',(1.,0.,0.));
#30918=DIRECTION('',(0.,0.,-1.));
#30919=DIRECTION('center_axis',(1.,0.,0.));
#30920=DIRECTION('ref_axis',(0.,-1.,0.));
#30921=DIRECTION('center_axis',(1.,0.,0.));
#30922=DIRECTION('ref_axis',(0.,1.,0.));
#30923=DIRECTION('',(0.,-1.,0.));
#30924=DIRECTION('',(0.,0.,-1.));
#30925=DIRECTION('center_axis',(0.,-1.,0.));
#30926=DIRECTION('ref_axis',(-1.,0.,0.));
#30927=DIRECTION('',(-1.,0.,0.));
#30928=DIRECTION('',(-1.,0.,0.));
#30929=DIRECTION('',(0.,0.,-1.));
#30930=DIRECTION('center_axis',(-1.,0.,0.));
#30931=DIRECTION('ref_axis',(0.,1.,0.));
#30932=DIRECTION('center_axis',(-1.,0.,0.));
#30933=DIRECTION('ref_axis',(0.,1.,0.));
#30934=DIRECTION('',(0.,1.,0.));
#30935=DIRECTION('center_axis',(0.,0.,-1.));
#30936=DIRECTION('ref_axis',(-1.,0.,0.));
#30937=DIRECTION('center_axis',(0.,1.,0.));
#30938=DIRECTION('ref_axis',(1.,0.,0.));
#30939=DIRECTION('',(1.,0.,0.));
#30940=DIRECTION('',(0.,0.,-1.));
#30941=DIRECTION('',(1.,0.,0.));
#30942=DIRECTION('',(0.,0.,-1.));
#30943=DIRECTION('center_axis',(1.,0.,0.));
#30944=DIRECTION('ref_axis',(0.,-1.,0.));
#30945=DIRECTION('center_axis',(1.,0.,0.));
#30946=DIRECTION('ref_axis',(0.,1.,0.));
#30947=DIRECTION('',(0.,-1.,0.));
#30948=DIRECTION('',(0.,0.,-1.));
#30949=DIRECTION('center_axis',(0.,-1.,0.));
#30950=DIRECTION('ref_axis',(-1.,0.,0.));
#30951=DIRECTION('',(-1.,0.,0.));
#30952=DIRECTION('',(-1.,0.,0.));
#30953=DIRECTION('',(0.,0.,-1.));
#30954=DIRECTION('center_axis',(-1.,0.,0.));
#30955=DIRECTION('ref_axis',(0.,1.,0.));
#30956=DIRECTION('center_axis',(-1.,0.,0.));
#30957=DIRECTION('ref_axis',(0.,1.,0.));
#30958=DIRECTION('',(0.,1.,0.));
#30959=DIRECTION('center_axis',(0.,0.,-1.));
#30960=DIRECTION('ref_axis',(-1.,0.,0.));
#30961=DIRECTION('center_axis',(0.,1.,0.));
#30962=DIRECTION('ref_axis',(1.,0.,0.));
#30963=DIRECTION('',(1.,0.,0.));
#30964=DIRECTION('',(0.,0.,-1.));
#30965=DIRECTION('',(1.,0.,0.));
#30966=DIRECTION('',(0.,0.,-1.));
#30967=DIRECTION('center_axis',(1.,0.,0.));
#30968=DIRECTION('ref_axis',(0.,-1.,0.));
#30969=DIRECTION('center_axis',(1.,0.,0.));
#30970=DIRECTION('ref_axis',(0.,1.,0.));
#30971=DIRECTION('',(0.,-1.,0.));
#30972=DIRECTION('',(0.,0.,-1.));
#30973=DIRECTION('center_axis',(0.,-1.,0.));
#30974=DIRECTION('ref_axis',(-1.,0.,0.));
#30975=DIRECTION('',(-1.,0.,0.));
#30976=DIRECTION('',(-1.,0.,0.));
#30977=DIRECTION('',(0.,0.,-1.));
#30978=DIRECTION('center_axis',(-1.,0.,0.));
#30979=DIRECTION('ref_axis',(0.,1.,0.));
#30980=DIRECTION('center_axis',(-1.,0.,0.));
#30981=DIRECTION('ref_axis',(0.,1.,0.));
#30982=DIRECTION('',(0.,1.,0.));
#30983=DIRECTION('center_axis',(0.,0.,-1.));
#30984=DIRECTION('ref_axis',(-1.,0.,0.));
#30985=DIRECTION('center_axis',(0.,1.,0.));
#30986=DIRECTION('ref_axis',(1.,0.,0.));
#30987=DIRECTION('',(1.,0.,0.));
#30988=DIRECTION('',(0.,0.,-1.));
#30989=DIRECTION('',(1.,0.,0.));
#30990=DIRECTION('',(0.,0.,-1.));
#30991=DIRECTION('center_axis',(1.,0.,0.));
#30992=DIRECTION('ref_axis',(0.,-1.,0.));
#30993=DIRECTION('center_axis',(1.,0.,0.));
#30994=DIRECTION('ref_axis',(0.,1.,0.));
#30995=DIRECTION('',(0.,-1.,0.));
#30996=DIRECTION('',(0.,0.,-1.));
#30997=DIRECTION('center_axis',(0.,-1.,0.));
#30998=DIRECTION('ref_axis',(-1.,0.,0.));
#30999=DIRECTION('',(-1.,0.,0.));
#31000=DIRECTION('',(-1.,0.,0.));
#31001=DIRECTION('',(0.,0.,-1.));
#31002=DIRECTION('center_axis',(-1.,0.,0.));
#31003=DIRECTION('ref_axis',(0.,1.,0.));
#31004=DIRECTION('center_axis',(-1.,0.,0.));
#31005=DIRECTION('ref_axis',(0.,1.,0.));
#31006=DIRECTION('',(0.,1.,0.));
#31007=DIRECTION('center_axis',(0.,0.,-1.));
#31008=DIRECTION('ref_axis',(-1.,0.,0.));
#31009=DIRECTION('center_axis',(0.,1.,0.));
#31010=DIRECTION('ref_axis',(1.,0.,0.));
#31011=DIRECTION('',(1.,0.,0.));
#31012=DIRECTION('',(0.,0.,-1.));
#31013=DIRECTION('',(1.,0.,0.));
#31014=DIRECTION('',(0.,0.,-1.));
#31015=DIRECTION('center_axis',(1.,0.,0.));
#31016=DIRECTION('ref_axis',(0.,-1.,0.));
#31017=DIRECTION('center_axis',(1.,0.,0.));
#31018=DIRECTION('ref_axis',(0.,1.,0.));
#31019=DIRECTION('',(0.,-1.,0.));
#31020=DIRECTION('',(0.,0.,-1.));
#31021=DIRECTION('center_axis',(0.,-1.,0.));
#31022=DIRECTION('ref_axis',(-1.,0.,0.));
#31023=DIRECTION('',(-1.,0.,0.));
#31024=DIRECTION('',(-1.,0.,0.));
#31025=DIRECTION('',(0.,0.,-1.));
#31026=DIRECTION('center_axis',(-1.,0.,0.));
#31027=DIRECTION('ref_axis',(0.,1.,0.));
#31028=DIRECTION('center_axis',(-1.,0.,0.));
#31029=DIRECTION('ref_axis',(0.,1.,0.));
#31030=DIRECTION('',(0.,1.,0.));
#31031=DIRECTION('center_axis',(0.,0.,-1.));
#31032=DIRECTION('ref_axis',(-1.,0.,0.));
#31033=DIRECTION('center_axis',(0.,1.,0.));
#31034=DIRECTION('ref_axis',(1.,0.,0.));
#31035=DIRECTION('',(1.,0.,0.));
#31036=DIRECTION('',(0.,0.,-1.));
#31037=DIRECTION('',(1.,0.,0.));
#31038=DIRECTION('',(0.,0.,-1.));
#31039=DIRECTION('center_axis',(1.,0.,0.));
#31040=DIRECTION('ref_axis',(0.,-1.,0.));
#31041=DIRECTION('center_axis',(1.,0.,0.));
#31042=DIRECTION('ref_axis',(0.,1.,0.));
#31043=DIRECTION('',(0.,-1.,0.));
#31044=DIRECTION('',(0.,0.,-1.));
#31045=DIRECTION('center_axis',(0.,-1.,0.));
#31046=DIRECTION('ref_axis',(-1.,0.,0.));
#31047=DIRECTION('',(-1.,0.,0.));
#31048=DIRECTION('',(-1.,0.,0.));
#31049=DIRECTION('',(0.,0.,-1.));
#31050=DIRECTION('center_axis',(-1.,0.,0.));
#31051=DIRECTION('ref_axis',(0.,1.,0.));
#31052=DIRECTION('center_axis',(-1.,0.,0.));
#31053=DIRECTION('ref_axis',(0.,1.,0.));
#31054=DIRECTION('',(0.,1.,0.));
#31055=DIRECTION('center_axis',(0.,0.,-1.));
#31056=DIRECTION('ref_axis',(-1.,0.,0.));
#31057=DIRECTION('center_axis',(0.,1.,0.));
#31058=DIRECTION('ref_axis',(1.,0.,0.));
#31059=DIRECTION('',(1.,0.,0.));
#31060=DIRECTION('',(0.,0.,-1.));
#31061=DIRECTION('',(1.,0.,0.));
#31062=DIRECTION('',(0.,0.,-1.));
#31063=DIRECTION('center_axis',(1.,0.,0.));
#31064=DIRECTION('ref_axis',(0.,-1.,0.));
#31065=DIRECTION('center_axis',(1.,0.,0.));
#31066=DIRECTION('ref_axis',(0.,1.,0.));
#31067=DIRECTION('',(0.,-1.,0.));
#31068=DIRECTION('',(0.,0.,-1.));
#31069=DIRECTION('center_axis',(0.,-1.,0.));
#31070=DIRECTION('ref_axis',(-1.,0.,0.));
#31071=DIRECTION('',(-1.,0.,0.));
#31072=DIRECTION('',(-1.,0.,0.));
#31073=DIRECTION('',(0.,0.,-1.));
#31074=DIRECTION('center_axis',(-1.,0.,0.));
#31075=DIRECTION('ref_axis',(0.,1.,0.));
#31076=DIRECTION('center_axis',(-1.,0.,0.));
#31077=DIRECTION('ref_axis',(0.,1.,0.));
#31078=DIRECTION('',(0.,1.,0.));
#31079=DIRECTION('center_axis',(0.,0.,-1.));
#31080=DIRECTION('ref_axis',(-1.,0.,0.));
#31081=DIRECTION('center_axis',(0.,1.,0.));
#31082=DIRECTION('ref_axis',(1.,0.,0.));
#31083=DIRECTION('',(1.,0.,0.));
#31084=DIRECTION('',(0.,0.,-1.));
#31085=DIRECTION('',(1.,0.,0.));
#31086=DIRECTION('',(0.,0.,-1.));
#31087=DIRECTION('center_axis',(1.,0.,0.));
#31088=DIRECTION('ref_axis',(0.,-1.,0.));
#31089=DIRECTION('center_axis',(1.,0.,0.));
#31090=DIRECTION('ref_axis',(0.,1.,0.));
#31091=DIRECTION('',(0.,-1.,0.));
#31092=DIRECTION('',(0.,0.,-1.));
#31093=DIRECTION('center_axis',(0.,-1.,0.));
#31094=DIRECTION('ref_axis',(-1.,0.,0.));
#31095=DIRECTION('',(-1.,0.,0.));
#31096=DIRECTION('',(-1.,0.,0.));
#31097=DIRECTION('',(0.,0.,-1.));
#31098=DIRECTION('center_axis',(-1.,0.,0.));
#31099=DIRECTION('ref_axis',(0.,1.,0.));
#31100=DIRECTION('center_axis',(-1.,0.,0.));
#31101=DIRECTION('ref_axis',(0.,1.,0.));
#31102=DIRECTION('',(0.,1.,0.));
#31103=DIRECTION('center_axis',(0.,0.,-1.));
#31104=DIRECTION('ref_axis',(-1.,0.,0.));
#31105=DIRECTION('center_axis',(0.,1.,0.));
#31106=DIRECTION('ref_axis',(1.,0.,0.));
#31107=DIRECTION('',(1.,0.,0.));
#31108=DIRECTION('',(0.,0.,-1.));
#31109=DIRECTION('',(1.,0.,0.));
#31110=DIRECTION('',(0.,0.,-1.));
#31111=DIRECTION('center_axis',(1.,0.,0.));
#31112=DIRECTION('ref_axis',(0.,-1.,0.));
#31113=DIRECTION('center_axis',(1.,0.,0.));
#31114=DIRECTION('ref_axis',(0.,1.,0.));
#31115=DIRECTION('',(0.,-1.,0.));
#31116=DIRECTION('',(0.,0.,-1.));
#31117=DIRECTION('center_axis',(0.,-1.,0.));
#31118=DIRECTION('ref_axis',(-1.,0.,0.));
#31119=DIRECTION('',(-1.,0.,0.));
#31120=DIRECTION('',(-1.,0.,0.));
#31121=DIRECTION('',(0.,0.,-1.));
#31122=DIRECTION('center_axis',(-1.,0.,0.));
#31123=DIRECTION('ref_axis',(0.,1.,0.));
#31124=DIRECTION('center_axis',(-1.,0.,0.));
#31125=DIRECTION('ref_axis',(0.,1.,0.));
#31126=DIRECTION('',(0.,1.,0.));
#31127=DIRECTION('center_axis',(0.,0.,-1.));
#31128=DIRECTION('ref_axis',(-1.,0.,0.));
#31129=DIRECTION('center_axis',(0.,1.,0.));
#31130=DIRECTION('ref_axis',(1.,0.,0.));
#31131=DIRECTION('',(1.,0.,0.));
#31132=DIRECTION('',(0.,0.,-1.));
#31133=DIRECTION('',(1.,0.,0.));
#31134=DIRECTION('',(0.,0.,-1.));
#31135=DIRECTION('center_axis',(1.,0.,0.));
#31136=DIRECTION('ref_axis',(0.,-1.,0.));
#31137=DIRECTION('center_axis',(1.,0.,0.));
#31138=DIRECTION('ref_axis',(0.,1.,0.));
#31139=DIRECTION('',(0.,-1.,0.));
#31140=DIRECTION('',(0.,0.,-1.));
#31141=DIRECTION('center_axis',(0.,-1.,0.));
#31142=DIRECTION('ref_axis',(-1.,0.,0.));
#31143=DIRECTION('',(-1.,0.,0.));
#31144=DIRECTION('',(-1.,0.,0.));
#31145=DIRECTION('',(0.,0.,-1.));
#31146=DIRECTION('center_axis',(-1.,0.,0.));
#31147=DIRECTION('ref_axis',(0.,1.,0.));
#31148=DIRECTION('center_axis',(-1.,0.,0.));
#31149=DIRECTION('ref_axis',(0.,1.,0.));
#31150=DIRECTION('',(0.,1.,0.));
#31151=DIRECTION('center_axis',(0.,0.,-1.));
#31152=DIRECTION('ref_axis',(-1.,0.,0.));
#31153=DIRECTION('center_axis',(0.,1.,0.));
#31154=DIRECTION('ref_axis',(1.,0.,0.));
#31155=DIRECTION('',(1.,0.,0.));
#31156=DIRECTION('',(0.,0.,-1.));
#31157=DIRECTION('',(1.,0.,0.));
#31158=DIRECTION('',(0.,0.,-1.));
#31159=DIRECTION('center_axis',(1.,0.,0.));
#31160=DIRECTION('ref_axis',(0.,-1.,0.));
#31161=DIRECTION('center_axis',(1.,0.,0.));
#31162=DIRECTION('ref_axis',(0.,1.,0.));
#31163=DIRECTION('',(0.,-1.,0.));
#31164=DIRECTION('',(0.,0.,-1.));
#31165=DIRECTION('center_axis',(0.,-1.,0.));
#31166=DIRECTION('ref_axis',(-1.,0.,0.));
#31167=DIRECTION('',(-1.,0.,0.));
#31168=DIRECTION('',(-1.,0.,0.));
#31169=DIRECTION('',(0.,0.,-1.));
#31170=DIRECTION('center_axis',(-1.,0.,0.));
#31171=DIRECTION('ref_axis',(0.,1.,0.));
#31172=DIRECTION('center_axis',(-1.,0.,0.));
#31173=DIRECTION('ref_axis',(0.,1.,0.));
#31174=DIRECTION('',(0.,1.,0.));
#31175=DIRECTION('center_axis',(0.,0.,-1.));
#31176=DIRECTION('ref_axis',(-1.,0.,0.));
#31177=DIRECTION('center_axis',(0.,1.,0.));
#31178=DIRECTION('ref_axis',(1.,0.,0.));
#31179=DIRECTION('',(1.,0.,0.));
#31180=DIRECTION('',(0.,0.,-1.));
#31181=DIRECTION('',(1.,0.,0.));
#31182=DIRECTION('',(0.,0.,-1.));
#31183=DIRECTION('center_axis',(1.,0.,0.));
#31184=DIRECTION('ref_axis',(0.,-1.,0.));
#31185=DIRECTION('center_axis',(1.,0.,0.));
#31186=DIRECTION('ref_axis',(0.,1.,0.));
#31187=DIRECTION('',(0.,-1.,0.));
#31188=DIRECTION('',(0.,0.,-1.));
#31189=DIRECTION('center_axis',(0.,-1.,0.));
#31190=DIRECTION('ref_axis',(-1.,0.,0.));
#31191=DIRECTION('',(-1.,0.,0.));
#31192=DIRECTION('',(-1.,0.,0.));
#31193=DIRECTION('',(0.,0.,-1.));
#31194=DIRECTION('center_axis',(-1.,0.,0.));
#31195=DIRECTION('ref_axis',(0.,1.,0.));
#31196=DIRECTION('center_axis',(-1.,0.,0.));
#31197=DIRECTION('ref_axis',(0.,1.,0.));
#31198=DIRECTION('',(0.,1.,0.));
#31199=DIRECTION('center_axis',(0.,0.,-1.));
#31200=DIRECTION('ref_axis',(-1.,0.,0.));
#31201=DIRECTION('center_axis',(0.,1.,0.));
#31202=DIRECTION('ref_axis',(1.,0.,0.));
#31203=DIRECTION('',(1.,0.,0.));
#31204=DIRECTION('',(0.,0.,-1.));
#31205=DIRECTION('',(1.,0.,0.));
#31206=DIRECTION('',(0.,0.,-1.));
#31207=DIRECTION('center_axis',(1.,0.,0.));
#31208=DIRECTION('ref_axis',(0.,-1.,0.));
#31209=DIRECTION('center_axis',(1.,0.,0.));
#31210=DIRECTION('ref_axis',(0.,1.,0.));
#31211=DIRECTION('',(0.,-1.,0.));
#31212=DIRECTION('',(0.,0.,-1.));
#31213=DIRECTION('center_axis',(0.,-1.,0.));
#31214=DIRECTION('ref_axis',(-1.,0.,0.));
#31215=DIRECTION('',(-1.,0.,0.));
#31216=DIRECTION('',(-1.,0.,0.));
#31217=DIRECTION('',(0.,0.,-1.));
#31218=DIRECTION('center_axis',(-1.,0.,0.));
#31219=DIRECTION('ref_axis',(0.,1.,0.));
#31220=DIRECTION('center_axis',(-1.,0.,0.));
#31221=DIRECTION('ref_axis',(0.,1.,0.));
#31222=DIRECTION('',(0.,1.,0.));
#31223=DIRECTION('center_axis',(0.,0.,-1.));
#31224=DIRECTION('ref_axis',(-1.,0.,0.));
#31225=DIRECTION('center_axis',(0.,1.,0.));
#31226=DIRECTION('ref_axis',(1.,0.,0.));
#31227=DIRECTION('',(1.,0.,0.));
#31228=DIRECTION('',(0.,0.,-1.));
#31229=DIRECTION('',(1.,0.,0.));
#31230=DIRECTION('',(0.,0.,-1.));
#31231=DIRECTION('center_axis',(1.,0.,0.));
#31232=DIRECTION('ref_axis',(0.,-1.,0.));
#31233=DIRECTION('center_axis',(1.,0.,0.));
#31234=DIRECTION('ref_axis',(0.,1.,0.));
#31235=DIRECTION('',(0.,-1.,0.));
#31236=DIRECTION('',(0.,0.,-1.));
#31237=DIRECTION('center_axis',(0.,-1.,0.));
#31238=DIRECTION('ref_axis',(-1.,0.,0.));
#31239=DIRECTION('',(-1.,0.,0.));
#31240=DIRECTION('',(-1.,0.,0.));
#31241=DIRECTION('',(0.,0.,-1.));
#31242=DIRECTION('center_axis',(-1.,0.,0.));
#31243=DIRECTION('ref_axis',(0.,1.,0.));
#31244=DIRECTION('center_axis',(-1.,0.,0.));
#31245=DIRECTION('ref_axis',(0.,1.,0.));
#31246=DIRECTION('',(0.,1.,0.));
#31247=DIRECTION('center_axis',(0.,0.,-1.));
#31248=DIRECTION('ref_axis',(-1.,0.,0.));
#31249=DIRECTION('center_axis',(0.,1.,0.));
#31250=DIRECTION('ref_axis',(1.,0.,0.));
#31251=DIRECTION('',(1.,0.,0.));
#31252=DIRECTION('',(0.,0.,-1.));
#31253=DIRECTION('',(1.,0.,0.));
#31254=DIRECTION('',(0.,0.,-1.));
#31255=DIRECTION('center_axis',(1.,0.,0.));
#31256=DIRECTION('ref_axis',(0.,-1.,0.));
#31257=DIRECTION('center_axis',(1.,0.,0.));
#31258=DIRECTION('ref_axis',(0.,1.,0.));
#31259=DIRECTION('',(0.,-1.,0.));
#31260=DIRECTION('',(0.,0.,-1.));
#31261=DIRECTION('center_axis',(0.,-1.,0.));
#31262=DIRECTION('ref_axis',(-1.,0.,0.));
#31263=DIRECTION('',(-1.,0.,0.));
#31264=DIRECTION('',(-1.,0.,0.));
#31265=DIRECTION('',(0.,0.,-1.));
#31266=DIRECTION('center_axis',(-1.,0.,0.));
#31267=DIRECTION('ref_axis',(0.,1.,0.));
#31268=DIRECTION('center_axis',(-1.,0.,0.));
#31269=DIRECTION('ref_axis',(0.,1.,0.));
#31270=DIRECTION('',(0.,1.,0.));
#31271=DIRECTION('center_axis',(0.,0.,-1.));
#31272=DIRECTION('ref_axis',(-1.,0.,0.));
#31273=DIRECTION('center_axis',(0.,1.,0.));
#31274=DIRECTION('ref_axis',(1.,0.,0.));
#31275=DIRECTION('',(1.,0.,0.));
#31276=DIRECTION('',(0.,0.,-1.));
#31277=DIRECTION('',(1.,0.,0.));
#31278=DIRECTION('',(0.,0.,-1.));
#31279=DIRECTION('center_axis',(1.,0.,0.));
#31280=DIRECTION('ref_axis',(0.,-1.,0.));
#31281=DIRECTION('center_axis',(1.,0.,0.));
#31282=DIRECTION('ref_axis',(0.,1.,0.));
#31283=DIRECTION('',(0.,-1.,0.));
#31284=DIRECTION('',(0.,0.,-1.));
#31285=DIRECTION('center_axis',(0.,-1.,0.));
#31286=DIRECTION('ref_axis',(-1.,0.,0.));
#31287=DIRECTION('',(-1.,0.,0.));
#31288=DIRECTION('',(-1.,0.,0.));
#31289=DIRECTION('',(0.,0.,-1.));
#31290=DIRECTION('center_axis',(-1.,0.,0.));
#31291=DIRECTION('ref_axis',(0.,1.,0.));
#31292=DIRECTION('center_axis',(-1.,0.,0.));
#31293=DIRECTION('ref_axis',(0.,1.,0.));
#31294=DIRECTION('',(0.,1.,0.));
#31295=DIRECTION('center_axis',(0.,0.,-1.));
#31296=DIRECTION('ref_axis',(-1.,0.,0.));
#31297=DIRECTION('center_axis',(0.,1.,0.));
#31298=DIRECTION('ref_axis',(1.,0.,0.));
#31299=DIRECTION('',(1.,0.,0.));
#31300=DIRECTION('',(0.,0.,-1.));
#31301=DIRECTION('',(1.,0.,0.));
#31302=DIRECTION('',(0.,0.,-1.));
#31303=DIRECTION('center_axis',(1.,0.,0.));
#31304=DIRECTION('ref_axis',(0.,-1.,0.));
#31305=DIRECTION('center_axis',(1.,0.,0.));
#31306=DIRECTION('ref_axis',(0.,1.,0.));
#31307=DIRECTION('',(0.,-1.,0.));
#31308=DIRECTION('',(0.,0.,-1.));
#31309=DIRECTION('center_axis',(0.,-1.,0.));
#31310=DIRECTION('ref_axis',(-1.,0.,0.));
#31311=DIRECTION('',(-1.,0.,0.));
#31312=DIRECTION('',(-1.,0.,0.));
#31313=DIRECTION('',(0.,0.,-1.));
#31314=DIRECTION('center_axis',(-1.,0.,0.));
#31315=DIRECTION('ref_axis',(0.,1.,0.));
#31316=DIRECTION('center_axis',(-1.,0.,0.));
#31317=DIRECTION('ref_axis',(0.,1.,0.));
#31318=DIRECTION('',(0.,1.,0.));
#31319=DIRECTION('center_axis',(0.,0.,-1.));
#31320=DIRECTION('ref_axis',(-1.,0.,0.));
#31321=DIRECTION('center_axis',(0.,1.,0.));
#31322=DIRECTION('ref_axis',(1.,0.,0.));
#31323=DIRECTION('',(-1.,0.,0.));
#31324=DIRECTION('',(0.,0.,-1.));
#31325=DIRECTION('',(-1.,0.,0.));
#31326=DIRECTION('',(0.,0.,-1.));
#31327=DIRECTION('center_axis',(0.,0.,-1.));
#31328=DIRECTION('ref_axis',(1.1842378929335E-14,1.,0.));
#31329=DIRECTION('center_axis',(0.,0.,1.));
#31330=DIRECTION('ref_axis',(1.1842378929335E-14,1.,0.));
#31331=DIRECTION('',(0.,0.,-1.));
#31332=DIRECTION('center_axis',(0.,-1.,0.));
#31333=DIRECTION('ref_axis',(-1.,0.,0.));
#31334=DIRECTION('',(1.,0.,0.));
#31335=DIRECTION('',(1.,0.,0.));
#31336=DIRECTION('',(0.,0.,-1.));
#31337=DIRECTION('center_axis',(0.,0.,-1.));
#31338=DIRECTION('ref_axis',(0.,-1.,0.));
#31339=DIRECTION('center_axis',(0.,0.,1.));
#31340=DIRECTION('ref_axis',(0.,-1.,0.));
#31341=DIRECTION('center_axis',(0.,0.,1.));
#31342=DIRECTION('ref_axis',(1.,0.,0.));
#31343=DIRECTION('center_axis',(1.,0.,0.));
#31344=DIRECTION('ref_axis',(0.,1.,0.));
#31345=DIRECTION('center_axis',(1.,0.,0.));
#31346=DIRECTION('ref_axis',(0.,0.,-1.));
#31347=DIRECTION('',(-1.,0.,0.));
#31348=DIRECTION('center_axis',(1.,0.,0.));
#31349=DIRECTION('ref_axis',(0.,0.,-1.));
#31350=DIRECTION('center_axis',(-1.,0.,0.));
#31351=DIRECTION('ref_axis',(0.,0.,1.));
#31352=DIRECTION('center_axis',(1.,0.,0.));
#31353=DIRECTION('ref_axis',(0.,0.,-1.));
#31354=DIRECTION('center_axis',(1.,0.,0.));
#31355=DIRECTION('ref_axis',(0.,1.,0.));
#31356=DIRECTION('center_axis',(1.,0.,0.));
#31357=DIRECTION('ref_axis',(0.,0.,-1.));
#31358=DIRECTION('',(-0.707106781186546,0.707106781186549,8.65956056235495E-17));
#31359=DIRECTION('center_axis',(1.,0.,0.));
#31360=DIRECTION('ref_axis',(0.,1.,0.));
#31361=DIRECTION('',(-1.,0.,0.));
#31362=DIRECTION('center_axis',(1.,0.,0.));
#31363=DIRECTION('ref_axis',(0.,1.,0.));
#31364=DIRECTION('',(-0.697985354304537,0.71611203395584,8.7698431021492E-17));
#31365=DIRECTION('center_axis',(1.,0.,0.));
#31366=DIRECTION('ref_axis',(0.,0.,-1.));
#31367=DIRECTION('center_axis',(1.,0.,0.));
#31368=DIRECTION('ref_axis',(0.,1.,0.));
#31369=DIRECTION('',(-0.999662950030635,0.0259612468122956,3.17933578105522E-18));
#31370=DIRECTION('center_axis',(1.,0.,0.));
#31371=DIRECTION('ref_axis',(0.,0.,-1.));
#31372=DIRECTION('center_axis',(1.,0.,0.));
#31373=DIRECTION('ref_axis',(0.,0.,-1.));
#31374=DIRECTION('center_axis',(1.,0.,0.));
#31375=DIRECTION('ref_axis',(0.,0.,-1.));
#31376=DIRECTION('center_axis',(1.,0.,0.));
#31377=DIRECTION('ref_axis',(0.,1.,0.));
#31378=DIRECTION('',(-1.,0.,0.));
#31379=DIRECTION('center_axis',(1.,0.,0.));
#31380=DIRECTION('ref_axis',(0.,0.,-1.));
#31381=DIRECTION('center_axis',(-1.,0.,0.));
#31382=DIRECTION('ref_axis',(0.,0.,1.));
#39436=CARTESIAN_POINT('',(0.,0.,0.));
#39437=CARTESIAN_POINT('Origin',(38.9767641234007,0.,26.5));
#39438=CARTESIAN_POINT('',(39.,3.05,26.5));
#39439=CARTESIAN_POINT('Origin',(39.,0.,26.5));
#39440=CARTESIAN_POINT('',(38.9535282468013,3.11844928601987,26.5));
#39441=CARTESIAN_POINT('',(38.9767641234007,3.08422464300993,26.5));
#39442=CARTESIAN_POINT('',(38.9535282468013,-3.11844928601987,26.5));
#39443=CARTESIAN_POINT('Origin',(38.9535282468013,0.,26.5));
#39444=CARTESIAN_POINT('Origin',(38.9535282468013,0.,26.5));
#39445=CARTESIAN_POINT('Origin',(38.5,0.,26.5));
#39446=CARTESIAN_POINT('',(38.,-3.497,26.5));
#39447=CARTESIAN_POINT('',(38.5,-3.2985,26.5));
#39448=CARTESIAN_POINT('Origin',(38.,0.,26.5));
#39449=CARTESIAN_POINT('Origin',(39.,1.64335,26.5));
#39450=CARTESIAN_POINT('',(39.,-1.64335,26.5));
#39451=CARTESIAN_POINT('Origin',(39.,0.,26.5));
#39452=CARTESIAN_POINT('Origin',(27.97,0.2,30.097));
#39453=CARTESIAN_POINT('',(27.97,0.2,29.9912761277218));
#39454=CARTESIAN_POINT('',(28.03,0.2,29.9912761277218));
#39455=CARTESIAN_POINT('',(24.05,0.2,29.9912761277218));
#39456=CARTESIAN_POINT('',(27.97,0.2,29.957));
#39457=CARTESIAN_POINT('',(27.97,0.2,30.097));
#39458=CARTESIAN_POINT('',(28.03,0.2,29.957));
#39459=CARTESIAN_POINT('',(28.03,0.2,29.957));
#39460=CARTESIAN_POINT('',(28.03,0.2,30.097));
#39461=CARTESIAN_POINT('Origin',(28.03,0.2,30.097));
#39462=CARTESIAN_POINT('',(28.03,-0.2,29.9912761277218));
#39463=CARTESIAN_POINT('Origin',(28.03,0.,26.5));
#39464=CARTESIAN_POINT('',(28.03,-0.2,29.957));
#39465=CARTESIAN_POINT('',(28.03,-0.2,29.957));
#39466=CARTESIAN_POINT('',(28.03,-0.2,30.097));
#39467=CARTESIAN_POINT('Origin',(28.03,-0.2,30.097));
#39468=CARTESIAN_POINT('',(27.97,-0.2,29.9912761277218));
#39469=CARTESIAN_POINT('',(24.05,-0.2,29.9912761277218));
#39470=CARTESIAN_POINT('',(27.97,-0.2,29.957));
#39471=CARTESIAN_POINT('',(27.97,-0.2,29.957));
#39472=CARTESIAN_POINT('',(27.97,-0.2,30.097));
#39473=CARTESIAN_POINT('Origin',(27.97,-0.2,30.097));
#39474=CARTESIAN_POINT('Origin',(27.97,0.,26.5));
#39475=CARTESIAN_POINT('',(27.97,0.2,29.957));
#39476=CARTESIAN_POINT('Origin',(28.,0.,29.957));
#39477=CARTESIAN_POINT('Origin',(28.97,0.2,30.097));
#39478=CARTESIAN_POINT('',(28.97,0.2,29.9912761277218));
#39479=CARTESIAN_POINT('',(29.03,0.2,29.9912761277218));
#39480=CARTESIAN_POINT('',(24.05,0.2,29.9912761277218));
#39481=CARTESIAN_POINT('',(28.97,0.2,29.957));
#39482=CARTESIAN_POINT('',(28.97,0.2,30.097));
#39483=CARTESIAN_POINT('',(29.03,0.2,29.957));
#39484=CARTESIAN_POINT('',(29.03,0.2,29.957));
#39485=CARTESIAN_POINT('',(29.03,0.2,30.097));
#39486=CARTESIAN_POINT('Origin',(29.03,0.2,30.097));
#39487=CARTESIAN_POINT('',(29.03,-0.2,29.9912761277218));
#39488=CARTESIAN_POINT('Origin',(29.03,0.,26.5));
#39489=CARTESIAN_POINT('',(29.03,-0.2,29.957));
#39490=CARTESIAN_POINT('',(29.03,-0.2,29.957));
#39491=CARTESIAN_POINT('',(29.03,-0.2,30.097));
#39492=CARTESIAN_POINT('Origin',(29.03,-0.2,30.097));
#39493=CARTESIAN_POINT('',(28.97,-0.2,29.9912761277218));
#39494=CARTESIAN_POINT('',(24.05,-0.2,29.9912761277218));
#39495=CARTESIAN_POINT('',(28.97,-0.2,29.957));
#39496=CARTESIAN_POINT('',(28.97,-0.2,29.957));
#39497=CARTESIAN_POINT('',(28.97,-0.2,30.097));
#39498=CARTESIAN_POINT('Origin',(28.97,-0.2,30.097));
#39499=CARTESIAN_POINT('Origin',(28.97,0.,26.5));
#39500=CARTESIAN_POINT('',(28.97,0.2,29.957));
#39501=CARTESIAN_POINT('Origin',(29.,0.,29.957));
#39502=CARTESIAN_POINT('Origin',(29.97,0.2,30.097));
#39503=CARTESIAN_POINT('',(29.97,0.2,29.9912761277218));
#39504=CARTESIAN_POINT('',(30.03,0.2,29.9912761277218));
#39505=CARTESIAN_POINT('',(24.05,0.2,29.9912761277218));
#39506=CARTESIAN_POINT('',(29.97,0.2,29.957));
#39507=CARTESIAN_POINT('',(29.97,0.2,30.097));
#39508=CARTESIAN_POINT('',(30.03,0.2,29.957));
#39509=CARTESIAN_POINT('',(30.03,0.2,29.957));
#39510=CARTESIAN_POINT('',(30.03,0.2,30.097));
#39511=CARTESIAN_POINT('Origin',(30.03,0.2,30.097));
#39512=CARTESIAN_POINT('',(30.03,-0.2,29.9912761277218));
#39513=CARTESIAN_POINT('Origin',(30.03,0.,26.5));
#39514=CARTESIAN_POINT('',(30.03,-0.2,29.957));
#39515=CARTESIAN_POINT('',(30.03,-0.2,29.957));
#39516=CARTESIAN_POINT('',(30.03,-0.2,30.097));
#39517=CARTESIAN_POINT('Origin',(30.03,-0.2,30.097));
#39518=CARTESIAN_POINT('',(29.97,-0.2,29.9912761277218));
#39519=CARTESIAN_POINT('',(24.05,-0.2,29.9912761277218));
#39520=CARTESIAN_POINT('',(29.97,-0.2,29.957));
#39521=CARTESIAN_POINT('',(29.97,-0.2,29.957));
#39522=CARTESIAN_POINT('',(29.97,-0.2,30.097));
#39523=CARTESIAN_POINT('Origin',(29.97,-0.2,30.097));
#39524=CARTESIAN_POINT('Origin',(29.97,0.,26.5));
#39525=CARTESIAN_POINT('',(29.97,0.2,29.957));
#39526=CARTESIAN_POINT('Origin',(30.,0.,29.957));
#39527=CARTESIAN_POINT('Origin',(30.97,0.2,30.097));
#39528=CARTESIAN_POINT('',(30.97,0.2,29.9912761277218));
#39529=CARTESIAN_POINT('',(31.03,0.2,29.9912761277218));
#39530=CARTESIAN_POINT('',(24.05,0.2,29.9912761277218));
#39531=CARTESIAN_POINT('',(30.97,0.2,29.957));
#39532=CARTESIAN_POINT('',(30.97,0.2,30.097));
#39533=CARTESIAN_POINT('',(31.03,0.2,29.957));
#39534=CARTESIAN_POINT('',(31.03,0.2,29.957));
#39535=CARTESIAN_POINT('',(31.03,0.2,30.097));
#39536=CARTESIAN_POINT('Origin',(31.03,0.2,30.097));
#39537=CARTESIAN_POINT('',(31.03,-0.2,29.9912761277218));
#39538=CARTESIAN_POINT('Origin',(31.03,0.,26.5));
#39539=CARTESIAN_POINT('',(31.03,-0.2,29.957));
#39540=CARTESIAN_POINT('',(31.03,-0.2,29.957));
#39541=CARTESIAN_POINT('',(31.03,-0.2,30.097));
#39542=CARTESIAN_POINT('Origin',(31.03,-0.2,30.097));
#39543=CARTESIAN_POINT('',(30.97,-0.2,29.9912761277218));
#39544=CARTESIAN_POINT('',(24.05,-0.2,29.9912761277218));
#39545=CARTESIAN_POINT('',(30.97,-0.2,29.957));
#39546=CARTESIAN_POINT('',(30.97,-0.2,29.957));
#39547=CARTESIAN_POINT('',(30.97,-0.2,30.097));
#39548=CARTESIAN_POINT('Origin',(30.97,-0.2,30.097));
#39549=CARTESIAN_POINT('Origin',(30.97,0.,26.5));
#39550=CARTESIAN_POINT('',(30.97,0.2,29.957));
#39551=CARTESIAN_POINT('Origin',(31.,0.,29.957));
#39552=CARTESIAN_POINT('Origin',(31.97,0.2,30.097));
#39553=CARTESIAN_POINT('',(31.97,0.2,29.9912761277218));
#39554=CARTESIAN_POINT('',(32.03,0.2,29.9912761277218));
#39555=CARTESIAN_POINT('',(24.05,0.2,29.9912761277218));
#39556=CARTESIAN_POINT('',(31.97,0.2,29.957));
#39557=CARTESIAN_POINT('',(31.97,0.2,30.097));
#39558=CARTESIAN_POINT('',(32.03,0.2,29.957));
#39559=CARTESIAN_POINT('',(32.03,0.2,29.957));
#39560=CARTESIAN_POINT('',(32.03,0.2,30.097));
#39561=CARTESIAN_POINT('Origin',(32.03,0.2,30.097));
#39562=CARTESIAN_POINT('',(32.03,-0.2,29.9912761277218));
#39563=CARTESIAN_POINT('Origin',(32.03,0.,26.5));
#39564=CARTESIAN_POINT('',(32.03,-0.2,29.957));
#39565=CARTESIAN_POINT('',(32.03,-0.2,29.957));
#39566=CARTESIAN_POINT('',(32.03,-0.2,30.097));
#39567=CARTESIAN_POINT('Origin',(32.03,-0.2,30.097));
#39568=CARTESIAN_POINT('',(31.97,-0.2,29.9912761277218));
#39569=CARTESIAN_POINT('',(24.05,-0.2,29.9912761277218));
#39570=CARTESIAN_POINT('',(31.97,-0.2,29.957));
#39571=CARTESIAN_POINT('',(31.97,-0.2,29.957));
#39572=CARTESIAN_POINT('',(31.97,-0.2,30.097));
#39573=CARTESIAN_POINT('Origin',(31.97,-0.2,30.097));
#39574=CARTESIAN_POINT('Origin',(31.97,0.,26.5));
#39575=CARTESIAN_POINT('',(31.97,0.2,29.957));
#39576=CARTESIAN_POINT('Origin',(32.,0.,29.957));
#39577=CARTESIAN_POINT('Origin',(32.47,0.35,30.097));
#39578=CARTESIAN_POINT('',(32.47,0.35,29.9794409033636));
#39579=CARTESIAN_POINT('',(32.53,0.35,29.9794409033636));
#39580=CARTESIAN_POINT('',(24.05,0.35,29.9794409033636));
#39581=CARTESIAN_POINT('',(32.47,0.35,29.957));
#39582=CARTESIAN_POINT('',(32.47,0.35,30.097));
#39583=CARTESIAN_POINT('',(32.53,0.35,29.957));
#39584=CARTESIAN_POINT('',(32.53,0.35,29.957));
#39585=CARTESIAN_POINT('',(32.53,0.35,30.097));
#39586=CARTESIAN_POINT('Origin',(32.53,0.35,30.097));
#39587=CARTESIAN_POINT('',(32.53,-0.35,29.9794409033636));
#39588=CARTESIAN_POINT('Origin',(32.53,0.,26.5));
#39589=CARTESIAN_POINT('',(32.53,-0.35,29.957));
#39590=CARTESIAN_POINT('',(32.53,-0.35,29.957));
#39591=CARTESIAN_POINT('',(32.53,-0.35,30.097));
#39592=CARTESIAN_POINT('Origin',(32.53,-0.35,30.097));
#39593=CARTESIAN_POINT('',(32.47,-0.35,29.9794409033636));
#39594=CARTESIAN_POINT('',(24.05,-0.35,29.9794409033636));
#39595=CARTESIAN_POINT('',(32.47,-0.35,29.957));
#39596=CARTESIAN_POINT('',(32.47,-0.35,29.957));
#39597=CARTESIAN_POINT('',(32.47,-0.35,30.097));
#39598=CARTESIAN_POINT('Origin',(32.47,-0.35,30.097));
#39599=CARTESIAN_POINT('Origin',(32.47,0.,26.5));
#39600=CARTESIAN_POINT('',(32.47,0.35,29.957));
#39601=CARTESIAN_POINT('Origin',(32.5,0.,29.957));
#39602=CARTESIAN_POINT('Origin',(33.47,0.35,30.097));
#39603=CARTESIAN_POINT('',(33.47,0.35,29.9794409033636));
#39604=CARTESIAN_POINT('',(33.53,0.35,29.9794409033636));
#39605=CARTESIAN_POINT('',(24.05,0.35,29.9794409033636));
#39606=CARTESIAN_POINT('',(33.47,0.35,29.957));
#39607=CARTESIAN_POINT('',(33.47,0.35,30.097));
#39608=CARTESIAN_POINT('',(33.53,0.35,29.957));
#39609=CARTESIAN_POINT('',(33.53,0.35,29.957));
#39610=CARTESIAN_POINT('',(33.53,0.35,30.097));
#39611=CARTESIAN_POINT('Origin',(33.53,0.35,30.097));
#39612=CARTESIAN_POINT('',(33.53,-0.35,29.9794409033636));
#39613=CARTESIAN_POINT('Origin',(33.53,0.,26.5));
#39614=CARTESIAN_POINT('',(33.53,-0.35,29.957));
#39615=CARTESIAN_POINT('',(33.53,-0.35,29.957));
#39616=CARTESIAN_POINT('',(33.53,-0.35,30.097));
#39617=CARTESIAN_POINT('Origin',(33.53,-0.35,30.097));
#39618=CARTESIAN_POINT('',(33.47,-0.35,29.9794409033636));
#39619=CARTESIAN_POINT('',(24.05,-0.35,29.9794409033636));
#39620=CARTESIAN_POINT('',(33.47,-0.35,29.957));
#39621=CARTESIAN_POINT('',(33.47,-0.35,29.957));
#39622=CARTESIAN_POINT('',(33.47,-0.35,30.097));
#39623=CARTESIAN_POINT('Origin',(33.47,-0.35,30.097));
#39624=CARTESIAN_POINT('Origin',(33.47,0.,26.5));
#39625=CARTESIAN_POINT('',(33.47,0.35,29.957));
#39626=CARTESIAN_POINT('Origin',(33.5,0.,29.957));
#39627=CARTESIAN_POINT('Origin',(34.47,0.35,30.097));
#39628=CARTESIAN_POINT('',(34.47,0.35,29.9794409033636));
#39629=CARTESIAN_POINT('',(34.53,0.35,29.9794409033636));
#39630=CARTESIAN_POINT('',(24.05,0.35,29.9794409033636));
#39631=CARTESIAN_POINT('',(34.47,0.35,29.957));
#39632=CARTESIAN_POINT('',(34.47,0.35,30.097));
#39633=CARTESIAN_POINT('',(34.53,0.35,29.957));
#39634=CARTESIAN_POINT('',(34.53,0.35,29.957));
#39635=CARTESIAN_POINT('',(34.53,0.35,30.097));
#39636=CARTESIAN_POINT('Origin',(34.53,0.35,30.097));
#39637=CARTESIAN_POINT('',(34.53,-0.35,29.9794409033636));
#39638=CARTESIAN_POINT('Origin',(34.53,0.,26.5));
#39639=CARTESIAN_POINT('',(34.53,-0.35,29.957));
#39640=CARTESIAN_POINT('',(34.53,-0.35,29.957));
#39641=CARTESIAN_POINT('',(34.53,-0.35,30.097));
#39642=CARTESIAN_POINT('Origin',(34.53,-0.35,30.097));
#39643=CARTESIAN_POINT('',(34.47,-0.35,29.9794409033636));
#39644=CARTESIAN_POINT('',(24.05,-0.35,29.9794409033636));
#39645=CARTESIAN_POINT('',(34.47,-0.35,29.957));
#39646=CARTESIAN_POINT('',(34.47,-0.35,29.957));
#39647=CARTESIAN_POINT('',(34.47,-0.35,30.097));
#39648=CARTESIAN_POINT('Origin',(34.47,-0.35,30.097));
#39649=CARTESIAN_POINT('Origin',(34.47,0.,26.5));
#39650=CARTESIAN_POINT('',(34.47,0.35,29.957));
#39651=CARTESIAN_POINT('Origin',(34.5,0.,29.957));
#39652=CARTESIAN_POINT('Origin',(35.47,0.35,30.097));
#39653=CARTESIAN_POINT('',(35.47,0.35,29.9794409033636));
#39654=CARTESIAN_POINT('',(35.53,0.35,29.9794409033636));
#39655=CARTESIAN_POINT('',(24.05,0.35,29.9794409033636));
#39656=CARTESIAN_POINT('',(35.47,0.35,29.957));
#39657=CARTESIAN_POINT('',(35.47,0.35,30.097));
#39658=CARTESIAN_POINT('',(35.53,0.35,29.957));
#39659=CARTESIAN_POINT('',(35.53,0.35,29.957));
#39660=CARTESIAN_POINT('',(35.53,0.35,30.097));
#39661=CARTESIAN_POINT('Origin',(35.53,0.35,30.097));
#39662=CARTESIAN_POINT('',(35.53,-0.35,29.9794409033636));
#39663=CARTESIAN_POINT('Origin',(35.53,0.,26.5));
#39664=CARTESIAN_POINT('',(35.53,-0.35,29.957));
#39665=CARTESIAN_POINT('',(35.53,-0.35,29.957));
#39666=CARTESIAN_POINT('',(35.53,-0.35,30.097));
#39667=CARTESIAN_POINT('Origin',(35.53,-0.35,30.097));
#39668=CARTESIAN_POINT('',(35.47,-0.35,29.9794409033636));
#39669=CARTESIAN_POINT('',(24.05,-0.35,29.9794409033636));
#39670=CARTESIAN_POINT('',(35.47,-0.35,29.957));
#39671=CARTESIAN_POINT('',(35.47,-0.35,29.957));
#39672=CARTESIAN_POINT('',(35.47,-0.35,30.097));
#39673=CARTESIAN_POINT('Origin',(35.47,-0.35,30.097));
#39674=CARTESIAN_POINT('Origin',(35.47,0.,26.5));
#39675=CARTESIAN_POINT('',(35.47,0.35,29.957));
#39676=CARTESIAN_POINT('Origin',(35.5,0.,29.957));
#39677=CARTESIAN_POINT('Origin',(36.47,0.35,30.097));
#39678=CARTESIAN_POINT('',(36.47,0.35,29.9794409033636));
#39679=CARTESIAN_POINT('',(36.53,0.35,29.9794409033636));
#39680=CARTESIAN_POINT('',(24.05,0.35,29.9794409033636));
#39681=CARTESIAN_POINT('',(36.47,0.35,29.957));
#39682=CARTESIAN_POINT('',(36.47,0.35,30.097));
#39683=CARTESIAN_POINT('',(36.53,0.35,29.957));
#39684=CARTESIAN_POINT('',(36.53,0.35,29.957));
#39685=CARTESIAN_POINT('',(36.53,0.35,30.097));
#39686=CARTESIAN_POINT('Origin',(36.53,0.35,30.097));
#39687=CARTESIAN_POINT('',(36.53,-0.35,29.9794409033636));
#39688=CARTESIAN_POINT('Origin',(36.53,0.,26.5));
#39689=CARTESIAN_POINT('',(36.53,-0.35,29.957));
#39690=CARTESIAN_POINT('',(36.53,-0.35,29.957));
#39691=CARTESIAN_POINT('',(36.53,-0.35,30.097));
#39692=CARTESIAN_POINT('Origin',(36.53,-0.35,30.097));
#39693=CARTESIAN_POINT('',(36.47,-0.35,29.9794409033636));
#39694=CARTESIAN_POINT('',(24.05,-0.35,29.9794409033636));
#39695=CARTESIAN_POINT('',(36.47,-0.35,29.957));
#39696=CARTESIAN_POINT('',(36.47,-0.35,29.957));
#39697=CARTESIAN_POINT('',(36.47,-0.35,30.097));
#39698=CARTESIAN_POINT('Origin',(36.47,-0.35,30.097));
#39699=CARTESIAN_POINT('Origin',(36.47,0.,26.5));
#39700=CARTESIAN_POINT('',(36.47,0.35,29.957));
#39701=CARTESIAN_POINT('Origin',(36.5,0.,29.957));
#39702=CARTESIAN_POINT('Origin',(36.97,0.2,30.097));
#39703=CARTESIAN_POINT('',(36.97,0.2,29.9912761277218));
#39704=CARTESIAN_POINT('',(37.03,0.2,29.9912761277218));
#39705=CARTESIAN_POINT('',(24.05,0.2,29.9912761277218));
#39706=CARTESIAN_POINT('',(36.97,0.2,29.957));
#39707=CARTESIAN_POINT('',(36.97,0.2,30.097));
#39708=CARTESIAN_POINT('',(37.03,0.2,29.957));
#39709=CARTESIAN_POINT('',(37.03,0.2,29.957));
#39710=CARTESIAN_POINT('',(37.03,0.2,30.097));
#39711=CARTESIAN_POINT('Origin',(37.03,0.2,30.097));
#39712=CARTESIAN_POINT('',(37.03,-0.2,29.9912761277218));
#39713=CARTESIAN_POINT('Origin',(37.03,0.,26.5));
#39714=CARTESIAN_POINT('',(37.03,-0.2,29.957));
#39715=CARTESIAN_POINT('',(37.03,-0.2,29.957));
#39716=CARTESIAN_POINT('',(37.03,-0.2,30.097));
#39717=CARTESIAN_POINT('Origin',(37.03,-0.2,30.097));
#39718=CARTESIAN_POINT('',(36.97,-0.2,29.9912761277218));
#39719=CARTESIAN_POINT('',(24.05,-0.2,29.9912761277218));
#39720=CARTESIAN_POINT('',(36.97,-0.2,29.957));
#39721=CARTESIAN_POINT('',(36.97,-0.2,29.957));
#39722=CARTESIAN_POINT('',(36.97,-0.2,30.097));
#39723=CARTESIAN_POINT('Origin',(36.97,-0.2,30.097));
#39724=CARTESIAN_POINT('Origin',(36.97,0.,26.5));
#39725=CARTESIAN_POINT('',(36.97,0.2,29.957));
#39726=CARTESIAN_POINT('Origin',(37.,0.,29.957));
#39727=CARTESIAN_POINT('Origin',(35.97,0.2,30.097));
#39728=CARTESIAN_POINT('',(35.97,0.2,29.9912761277218));
#39729=CARTESIAN_POINT('',(36.03,0.2,29.9912761277218));
#39730=CARTESIAN_POINT('',(24.05,0.2,29.9912761277218));
#39731=CARTESIAN_POINT('',(35.97,0.2,29.957));
#39732=CARTESIAN_POINT('',(35.97,0.2,30.097));
#39733=CARTESIAN_POINT('',(36.03,0.2,29.957));
#39734=CARTESIAN_POINT('',(36.03,0.2,29.957));
#39735=CARTESIAN_POINT('',(36.03,0.2,30.097));
#39736=CARTESIAN_POINT('Origin',(36.03,0.2,30.097));
#39737=CARTESIAN_POINT('',(36.03,-0.2,29.9912761277218));
#39738=CARTESIAN_POINT('Origin',(36.03,0.,26.5));
#39739=CARTESIAN_POINT('',(36.03,-0.2,29.957));
#39740=CARTESIAN_POINT('',(36.03,-0.2,29.957));
#39741=CARTESIAN_POINT('',(36.03,-0.2,30.097));
#39742=CARTESIAN_POINT('Origin',(36.03,-0.2,30.097));
#39743=CARTESIAN_POINT('',(35.97,-0.2,29.9912761277218));
#39744=CARTESIAN_POINT('',(24.05,-0.2,29.9912761277218));
#39745=CARTESIAN_POINT('',(35.97,-0.2,29.957));
#39746=CARTESIAN_POINT('',(35.97,-0.2,29.957));
#39747=CARTESIAN_POINT('',(35.97,-0.2,30.097));
#39748=CARTESIAN_POINT('Origin',(35.97,-0.2,30.097));
#39749=CARTESIAN_POINT('Origin',(35.97,0.,26.5));
#39750=CARTESIAN_POINT('',(35.97,0.2,29.957));
#39751=CARTESIAN_POINT('Origin',(36.,0.,29.957));
#39752=CARTESIAN_POINT('Origin',(34.97,0.2,30.097));
#39753=CARTESIAN_POINT('',(34.97,0.2,29.9912761277218));
#39754=CARTESIAN_POINT('',(35.03,0.2,29.9912761277218));
#39755=CARTESIAN_POINT('',(24.05,0.2,29.9912761277218));
#39756=CARTESIAN_POINT('',(34.97,0.2,29.957));
#39757=CARTESIAN_POINT('',(34.97,0.2,30.097));
#39758=CARTESIAN_POINT('',(35.03,0.2,29.957));
#39759=CARTESIAN_POINT('',(35.03,0.2,29.957));
#39760=CARTESIAN_POINT('',(35.03,0.2,30.097));
#39761=CARTESIAN_POINT('Origin',(35.03,0.2,30.097));
#39762=CARTESIAN_POINT('',(35.03,-0.2,29.9912761277218));
#39763=CARTESIAN_POINT('Origin',(35.03,0.,26.5));
#39764=CARTESIAN_POINT('',(35.03,-0.2,29.957));
#39765=CARTESIAN_POINT('',(35.03,-0.2,29.957));
#39766=CARTESIAN_POINT('',(35.03,-0.2,30.097));
#39767=CARTESIAN_POINT('Origin',(35.03,-0.2,30.097));
#39768=CARTESIAN_POINT('',(34.97,-0.2,29.9912761277218));
#39769=CARTESIAN_POINT('',(24.05,-0.2,29.9912761277218));
#39770=CARTESIAN_POINT('',(34.97,-0.2,29.957));
#39771=CARTESIAN_POINT('',(34.97,-0.2,29.957));
#39772=CARTESIAN_POINT('',(34.97,-0.2,30.097));
#39773=CARTESIAN_POINT('Origin',(34.97,-0.2,30.097));
#39774=CARTESIAN_POINT('Origin',(34.97,0.,26.5));
#39775=CARTESIAN_POINT('',(34.97,0.2,29.957));
#39776=CARTESIAN_POINT('Origin',(35.,0.,29.957));
#39777=CARTESIAN_POINT('Origin',(33.97,0.2,30.097));
#39778=CARTESIAN_POINT('',(33.97,0.2,29.9912761277218));
#39779=CARTESIAN_POINT('',(34.03,0.2,29.9912761277218));
#39780=CARTESIAN_POINT('',(24.05,0.2,29.9912761277218));
#39781=CARTESIAN_POINT('',(33.97,0.2,29.957));
#39782=CARTESIAN_POINT('',(33.97,0.2,30.097));
#39783=CARTESIAN_POINT('',(34.03,0.2,29.957));
#39784=CARTESIAN_POINT('',(34.03,0.2,29.957));
#39785=CARTESIAN_POINT('',(34.03,0.2,30.097));
#39786=CARTESIAN_POINT('Origin',(34.03,0.2,30.097));
#39787=CARTESIAN_POINT('',(34.03,-0.2,29.9912761277218));
#39788=CARTESIAN_POINT('Origin',(34.03,0.,26.5));
#39789=CARTESIAN_POINT('',(34.03,-0.2,29.957));
#39790=CARTESIAN_POINT('',(34.03,-0.2,29.957));
#39791=CARTESIAN_POINT('',(34.03,-0.2,30.097));
#39792=CARTESIAN_POINT('Origin',(34.03,-0.2,30.097));
#39793=CARTESIAN_POINT('',(33.97,-0.2,29.9912761277218));
#39794=CARTESIAN_POINT('',(24.05,-0.2,29.9912761277218));
#39795=CARTESIAN_POINT('',(33.97,-0.2,29.957));
#39796=CARTESIAN_POINT('',(33.97,-0.2,29.957));
#39797=CARTESIAN_POINT('',(33.97,-0.2,30.097));
#39798=CARTESIAN_POINT('Origin',(33.97,-0.2,30.097));
#39799=CARTESIAN_POINT('Origin',(33.97,0.,26.5));
#39800=CARTESIAN_POINT('',(33.97,0.2,29.957));
#39801=CARTESIAN_POINT('Origin',(34.,0.,29.957));
#39802=CARTESIAN_POINT('Origin',(32.97,0.2,30.097));
#39803=CARTESIAN_POINT('',(32.97,0.2,29.9912761277218));
#39804=CARTESIAN_POINT('',(33.03,0.2,29.9912761277218));
#39805=CARTESIAN_POINT('',(24.05,0.2,29.9912761277218));
#39806=CARTESIAN_POINT('',(32.97,0.2,29.957));
#39807=CARTESIAN_POINT('',(32.97,0.2,30.097));
#39808=CARTESIAN_POINT('',(33.03,0.2,29.957));
#39809=CARTESIAN_POINT('',(33.03,0.2,29.957));
#39810=CARTESIAN_POINT('',(33.03,0.2,30.097));
#39811=CARTESIAN_POINT('Origin',(33.03,0.2,30.097));
#39812=CARTESIAN_POINT('',(33.03,-0.2,29.9912761277218));
#39813=CARTESIAN_POINT('Origin',(33.03,0.,26.5));
#39814=CARTESIAN_POINT('',(33.03,-0.2,29.957));
#39815=CARTESIAN_POINT('',(33.03,-0.2,29.957));
#39816=CARTESIAN_POINT('',(33.03,-0.2,30.097));
#39817=CARTESIAN_POINT('Origin',(33.03,-0.2,30.097));
#39818=CARTESIAN_POINT('',(32.97,-0.2,29.9912761277218));
#39819=CARTESIAN_POINT('',(24.05,-0.2,29.9912761277218));
#39820=CARTESIAN_POINT('',(32.97,-0.2,29.957));
#39821=CARTESIAN_POINT('',(32.97,-0.2,29.957));
#39822=CARTESIAN_POINT('',(32.97,-0.2,30.097));
#39823=CARTESIAN_POINT('Origin',(32.97,-0.2,30.097));
#39824=CARTESIAN_POINT('Origin',(32.97,0.,26.5));
#39825=CARTESIAN_POINT('',(32.97,0.2,29.957));
#39826=CARTESIAN_POINT('Origin',(33.,0.,29.957));
#39827=CARTESIAN_POINT('Origin',(37.47,0.35,30.097));
#39828=CARTESIAN_POINT('',(37.47,0.35,29.9794409033636));
#39829=CARTESIAN_POINT('',(37.53,0.35,29.9794409033636));
#39830=CARTESIAN_POINT('',(24.05,0.35,29.9794409033636));
#39831=CARTESIAN_POINT('',(37.47,0.35,29.957));
#39832=CARTESIAN_POINT('',(37.47,0.35,30.097));
#39833=CARTESIAN_POINT('',(37.53,0.35,29.957));
#39834=CARTESIAN_POINT('',(37.53,0.35,29.957));
#39835=CARTESIAN_POINT('',(37.53,0.35,30.097));
#39836=CARTESIAN_POINT('Origin',(37.53,0.35,30.097));
#39837=CARTESIAN_POINT('',(37.53,-0.35,29.9794409033636));
#39838=CARTESIAN_POINT('Origin',(37.53,0.,26.5));
#39839=CARTESIAN_POINT('',(37.53,-0.35,29.957));
#39840=CARTESIAN_POINT('',(37.53,-0.35,29.957));
#39841=CARTESIAN_POINT('',(37.53,-0.35,30.097));
#39842=CARTESIAN_POINT('Origin',(37.53,-0.35,30.097));
#39843=CARTESIAN_POINT('',(37.47,-0.35,29.9794409033636));
#39844=CARTESIAN_POINT('',(24.05,-0.35,29.9794409033636));
#39845=CARTESIAN_POINT('',(37.47,-0.35,29.957));
#39846=CARTESIAN_POINT('',(37.47,-0.35,29.957));
#39847=CARTESIAN_POINT('',(37.47,-0.35,30.097));
#39848=CARTESIAN_POINT('Origin',(37.47,-0.35,30.097));
#39849=CARTESIAN_POINT('Origin',(37.47,0.,26.5));
#39850=CARTESIAN_POINT('',(37.47,0.35,29.957));
#39851=CARTESIAN_POINT('Origin',(37.5,0.,29.957));
#39852=CARTESIAN_POINT('Origin',(31.47,0.35,30.097));
#39853=CARTESIAN_POINT('',(31.47,0.35,29.9794409033636));
#39854=CARTESIAN_POINT('',(31.53,0.35,29.9794409033636));
#39855=CARTESIAN_POINT('',(24.05,0.35,29.9794409033636));
#39856=CARTESIAN_POINT('',(31.47,0.35,29.957));
#39857=CARTESIAN_POINT('',(31.47,0.35,30.097));
#39858=CARTESIAN_POINT('',(31.53,0.35,29.957));
#39859=CARTESIAN_POINT('',(31.53,0.35,29.957));
#39860=CARTESIAN_POINT('',(31.53,0.35,30.097));
#39861=CARTESIAN_POINT('Origin',(31.53,0.35,30.097));
#39862=CARTESIAN_POINT('',(31.53,-0.35,29.9794409033636));
#39863=CARTESIAN_POINT('Origin',(31.53,0.,26.5));
#39864=CARTESIAN_POINT('',(31.53,-0.35,29.957));
#39865=CARTESIAN_POINT('',(31.53,-0.35,29.957));
#39866=CARTESIAN_POINT('',(31.53,-0.35,30.097));
#39867=CARTESIAN_POINT('Origin',(31.53,-0.35,30.097));
#39868=CARTESIAN_POINT('',(31.47,-0.35,29.9794409033636));
#39869=CARTESIAN_POINT('',(24.05,-0.35,29.9794409033636));
#39870=CARTESIAN_POINT('',(31.47,-0.35,29.957));
#39871=CARTESIAN_POINT('',(31.47,-0.35,29.957));
#39872=CARTESIAN_POINT('',(31.47,-0.35,30.097));
#39873=CARTESIAN_POINT('Origin',(31.47,-0.35,30.097));
#39874=CARTESIAN_POINT('Origin',(31.47,0.,26.5));
#39875=CARTESIAN_POINT('',(31.47,0.35,29.957));
#39876=CARTESIAN_POINT('Origin',(31.5,0.,29.957));
#39877=CARTESIAN_POINT('Origin',(30.47,0.35,30.097));
#39878=CARTESIAN_POINT('',(30.47,0.35,29.9794409033636));
#39879=CARTESIAN_POINT('',(30.53,0.35,29.9794409033636));
#39880=CARTESIAN_POINT('',(24.05,0.35,29.9794409033636));
#39881=CARTESIAN_POINT('',(30.47,0.35,29.957));
#39882=CARTESIAN_POINT('',(30.47,0.35,30.097));
#39883=CARTESIAN_POINT('',(30.53,0.35,29.957));
#39884=CARTESIAN_POINT('',(30.53,0.35,29.957));
#39885=CARTESIAN_POINT('',(30.53,0.35,30.097));
#39886=CARTESIAN_POINT('Origin',(30.53,0.35,30.097));
#39887=CARTESIAN_POINT('',(30.53,-0.35,29.9794409033636));
#39888=CARTESIAN_POINT('Origin',(30.53,0.,26.5));
#39889=CARTESIAN_POINT('',(30.53,-0.35,29.957));
#39890=CARTESIAN_POINT('',(30.53,-0.35,29.957));
#39891=CARTESIAN_POINT('',(30.53,-0.35,30.097));
#39892=CARTESIAN_POINT('Origin',(30.53,-0.35,30.097));
#39893=CARTESIAN_POINT('',(30.47,-0.35,29.9794409033636));
#39894=CARTESIAN_POINT('',(24.05,-0.35,29.9794409033636));
#39895=CARTESIAN_POINT('',(30.47,-0.35,29.957));
#39896=CARTESIAN_POINT('',(30.47,-0.35,29.957));
#39897=CARTESIAN_POINT('',(30.47,-0.35,30.097));
#39898=CARTESIAN_POINT('Origin',(30.47,-0.35,30.097));
#39899=CARTESIAN_POINT('Origin',(30.47,0.,26.5));
#39900=CARTESIAN_POINT('',(30.47,0.35,29.957));
#39901=CARTESIAN_POINT('Origin',(30.5,0.,29.957));
#39902=CARTESIAN_POINT('Origin',(29.47,0.35,30.097));
#39903=CARTESIAN_POINT('',(29.47,0.35,29.9794409033636));
#39904=CARTESIAN_POINT('',(29.53,0.35,29.9794409033636));
#39905=CARTESIAN_POINT('',(24.05,0.35,29.9794409033636));
#39906=CARTESIAN_POINT('',(29.47,0.35,29.957));
#39907=CARTESIAN_POINT('',(29.47,0.35,30.097));
#39908=CARTESIAN_POINT('',(29.53,0.35,29.957));
#39909=CARTESIAN_POINT('',(29.53,0.35,29.957));
#39910=CARTESIAN_POINT('',(29.53,0.35,30.097));
#39911=CARTESIAN_POINT('Origin',(29.53,0.35,30.097));
#39912=CARTESIAN_POINT('',(29.53,-0.35,29.9794409033636));
#39913=CARTESIAN_POINT('Origin',(29.53,0.,26.5));
#39914=CARTESIAN_POINT('',(29.53,-0.35,29.957));
#39915=CARTESIAN_POINT('',(29.53,-0.35,29.957));
#39916=CARTESIAN_POINT('',(29.53,-0.35,30.097));
#39917=CARTESIAN_POINT('Origin',(29.53,-0.35,30.097));
#39918=CARTESIAN_POINT('',(29.47,-0.35,29.9794409033636));
#39919=CARTESIAN_POINT('',(24.05,-0.35,29.9794409033636));
#39920=CARTESIAN_POINT('',(29.47,-0.35,29.957));
#39921=CARTESIAN_POINT('',(29.47,-0.35,29.957));
#39922=CARTESIAN_POINT('',(29.47,-0.35,30.097));
#39923=CARTESIAN_POINT('Origin',(29.47,-0.35,30.097));
#39924=CARTESIAN_POINT('Origin',(29.47,0.,26.5));
#39925=CARTESIAN_POINT('',(29.47,0.35,29.957));
#39926=CARTESIAN_POINT('Origin',(29.5,0.,29.957));
#39927=CARTESIAN_POINT('Origin',(28.47,0.35,30.097));
#39928=CARTESIAN_POINT('',(28.47,0.35,29.9794409033636));
#39929=CARTESIAN_POINT('',(28.53,0.35,29.9794409033636));
#39930=CARTESIAN_POINT('',(24.05,0.35,29.9794409033636));
#39931=CARTESIAN_POINT('',(28.47,0.35,29.957));
#39932=CARTESIAN_POINT('',(28.47,0.35,30.097));
#39933=CARTESIAN_POINT('',(28.53,0.35,29.957));
#39934=CARTESIAN_POINT('',(28.53,0.35,29.957));
#39935=CARTESIAN_POINT('',(28.53,0.35,30.097));
#39936=CARTESIAN_POINT('Origin',(28.53,0.35,30.097));
#39937=CARTESIAN_POINT('',(28.53,-0.35,29.9794409033636));
#39938=CARTESIAN_POINT('Origin',(28.53,0.,26.5));
#39939=CARTESIAN_POINT('',(28.53,-0.35,29.957));
#39940=CARTESIAN_POINT('',(28.53,-0.35,29.957));
#39941=CARTESIAN_POINT('',(28.53,-0.35,30.097));
#39942=CARTESIAN_POINT('Origin',(28.53,-0.35,30.097));
#39943=CARTESIAN_POINT('',(28.47,-0.35,29.9794409033636));
#39944=CARTESIAN_POINT('',(24.05,-0.35,29.9794409033636));
#39945=CARTESIAN_POINT('',(28.47,-0.35,29.957));
#39946=CARTESIAN_POINT('',(28.47,-0.35,29.957));
#39947=CARTESIAN_POINT('',(28.47,-0.35,30.097));
#39948=CARTESIAN_POINT('Origin',(28.47,-0.35,30.097));
#39949=CARTESIAN_POINT('Origin',(28.47,0.,26.5));
#39950=CARTESIAN_POINT('',(28.47,0.35,29.957));
#39951=CARTESIAN_POINT('Origin',(28.5,0.,29.957));
#39952=CARTESIAN_POINT('Origin',(27.47,0.35,30.097));
#39953=CARTESIAN_POINT('',(27.47,0.35,29.9794409033636));
#39954=CARTESIAN_POINT('',(27.53,0.35,29.9794409033636));
#39955=CARTESIAN_POINT('',(24.05,0.35,29.9794409033636));
#39956=CARTESIAN_POINT('',(27.47,0.35,29.957));
#39957=CARTESIAN_POINT('',(27.47,0.35,30.097));
#39958=CARTESIAN_POINT('',(27.53,0.35,29.957));
#39959=CARTESIAN_POINT('',(27.53,0.35,29.957));
#39960=CARTESIAN_POINT('',(27.53,0.35,30.097));
#39961=CARTESIAN_POINT('Origin',(27.53,0.35,30.097));
#39962=CARTESIAN_POINT('',(27.53,-0.35,29.9794409033636));
#39963=CARTESIAN_POINT('Origin',(27.53,0.,26.5));
#39964=CARTESIAN_POINT('',(27.53,-0.35,29.957));
#39965=CARTESIAN_POINT('',(27.53,-0.35,29.957));
#39966=CARTESIAN_POINT('',(27.53,-0.35,30.097));
#39967=CARTESIAN_POINT('Origin',(27.53,-0.35,30.097));
#39968=CARTESIAN_POINT('',(27.47,-0.35,29.9794409033636));
#39969=CARTESIAN_POINT('',(24.05,-0.35,29.9794409033636));
#39970=CARTESIAN_POINT('',(27.47,-0.35,29.957));
#39971=CARTESIAN_POINT('',(27.47,-0.35,29.957));
#39972=CARTESIAN_POINT('',(27.47,-0.35,30.097));
#39973=CARTESIAN_POINT('Origin',(27.47,-0.35,30.097));
#39974=CARTESIAN_POINT('Origin',(27.47,0.,26.5));
#39975=CARTESIAN_POINT('',(27.47,0.35,29.957));
#39976=CARTESIAN_POINT('Origin',(27.5,0.,29.957));
#39977=CARTESIAN_POINT('Origin',(23.8,0.3,23.303));
#39978=CARTESIAN_POINT('',(35.2,0.3,23.0158919362339));
#39979=CARTESIAN_POINT('',(23.8,0.3,23.0158919362339));
#39980=CARTESIAN_POINT('',(24.05,0.3,23.0158919362339));
#39981=CARTESIAN_POINT('',(35.2,0.3,23.303));
#39982=CARTESIAN_POINT('',(35.2,0.3,23.303));
#39983=CARTESIAN_POINT('',(23.8,0.3,23.303));
#39984=CARTESIAN_POINT('',(35.2,0.3,23.303));
#39985=CARTESIAN_POINT('',(23.8,0.3,23.303));
#39986=CARTESIAN_POINT('Origin',(23.8,0.,23.303));
#39987=CARTESIAN_POINT('',(23.8,-0.3,23.0158919362339));
#39988=CARTESIAN_POINT('Ctrl Pts',(23.8,0.3,23.0158919362339));
#39989=CARTESIAN_POINT('Ctrl Pts',(23.7623114146691,0.3,23.0158919362339));
#39990=CARTESIAN_POINT('Ctrl Pts',(23.7221234046193,0.292464132564535,23.0152174188699));
#39991=CARTESIAN_POINT('Ctrl Pts',(23.6482151108805,0.261842283181441,23.0127828394877));
#39992=CARTESIAN_POINT('Ctrl Pts',(23.6144932470194,0.238757315731349,23.0110581162707));
#39993=CARTESIAN_POINT('Ctrl Pts',(23.5612427332329,0.185506801944792,23.0078219192499));
#39994=CARTESIAN_POINT('Ctrl Pts',(23.5381577277572,0.151784916482474,23.0060999692551));
#39995=CARTESIAN_POINT('Ctrl Pts',(23.5075358494518,0.0778765510139039,
23.0036717361649));
#39996=CARTESIAN_POINT('Ctrl Pts',(23.5,0.0376885160210923,23.003));
#39997=CARTESIAN_POINT('Ctrl Pts',(23.5,-0.0376885160210922,23.003));
#39998=CARTESIAN_POINT('Ctrl Pts',(23.5075358494518,-0.0778765510139039,
23.0036717361649));
#39999=CARTESIAN_POINT('Ctrl Pts',(23.5381577277572,-0.151784916482474,
23.0060999692551));
#40000=CARTESIAN_POINT('Ctrl Pts',(23.5612427332329,-0.185506801944792,
23.0078219192499));
#40001=CARTESIAN_POINT('Ctrl Pts',(23.6144932470194,-0.238757315731349,
23.0110581162707));
#40002=CARTESIAN_POINT('Ctrl Pts',(23.6482151108805,-0.261842283181441,
23.0127828394877));
#40003=CARTESIAN_POINT('Ctrl Pts',(23.7221234046193,-0.292464132564535,
23.0152174188699));
#40004=CARTESIAN_POINT('Ctrl Pts',(23.7623114146691,-0.299999999999999,
23.0158919362339));
#40005=CARTESIAN_POINT('Ctrl Pts',(23.8,-0.3,23.0158919362339));
#40006=CARTESIAN_POINT('',(23.8,-0.3,23.303));
#40007=CARTESIAN_POINT('Origin',(23.8,0.,23.303));
#40008=CARTESIAN_POINT('',(23.8,-0.3,23.303));
#40009=CARTESIAN_POINT('Origin',(35.2,-0.3,23.303));
#40010=CARTESIAN_POINT('',(35.2,-0.3,23.0158919362339));
#40011=CARTESIAN_POINT('',(24.05,-0.3,23.0158919362339));
#40012=CARTESIAN_POINT('',(35.2,-0.3,23.303));
#40013=CARTESIAN_POINT('',(23.8,-0.3,23.303));
#40014=CARTESIAN_POINT('',(35.2,-0.3,23.303));
#40015=CARTESIAN_POINT('Origin',(35.2,2.77555756156289E-17,23.303));
#40016=CARTESIAN_POINT('Ctrl Pts',(35.2,-0.3,23.0158919362339));
#40017=CARTESIAN_POINT('Ctrl Pts',(35.2376885853309,-0.3,23.0158919362339));
#40018=CARTESIAN_POINT('Ctrl Pts',(35.2778765953807,-0.292464132564536,
23.0152174188699));
#40019=CARTESIAN_POINT('Ctrl Pts',(35.3517848891195,-0.261842283181445,
23.0127828394877));
#40020=CARTESIAN_POINT('Ctrl Pts',(35.3855067529806,-0.238757315731349,
23.0110581162707));
#40021=CARTESIAN_POINT('Ctrl Pts',(35.4387572667671,-0.185506801944793,
23.0078219192499));
#40022=CARTESIAN_POINT('Ctrl Pts',(35.4618422722428,-0.151784916482478,
23.0060999692551));
#40023=CARTESIAN_POINT('Ctrl Pts',(35.4924641505482,-0.0778765510139092,
23.0036717361649));
#40024=CARTESIAN_POINT('Ctrl Pts',(35.5,-0.0376885160210925,23.003));
#40025=CARTESIAN_POINT('Ctrl Pts',(35.5,0.0376885160210923,23.003));
#40026=CARTESIAN_POINT('Ctrl Pts',(35.4924641505482,0.077876551013909,23.0036717361649));
#40027=CARTESIAN_POINT('Ctrl Pts',(35.4618422722428,0.151784916482478,23.0060999692551));
#40028=CARTESIAN_POINT('Ctrl Pts',(35.4387572667671,0.185506801944793,23.0078219192499));
#40029=CARTESIAN_POINT('Ctrl Pts',(35.3855067529806,0.238757315731349,23.0110581162707));
#40030=CARTESIAN_POINT('Ctrl Pts',(35.3517848891195,0.261842283181443,23.0127828394877));
#40031=CARTESIAN_POINT('Ctrl Pts',(35.2778765953807,0.292464132564536,23.0152174188699));
#40032=CARTESIAN_POINT('Ctrl Pts',(35.2376885853309,0.3,23.0158919362339));
#40033=CARTESIAN_POINT('Ctrl Pts',(35.2,0.3,23.0158919362339));
#40034=CARTESIAN_POINT('Origin',(35.2,2.77555756156289E-17,23.303));
#40035=CARTESIAN_POINT('Origin',(29.5,0.,23.303));
#40036=CARTESIAN_POINT('Origin',(12.5,0.,26.5));
#40037=CARTESIAN_POINT('',(15.,-2.,26.5));
#40038=CARTESIAN_POINT('Origin',(15.,0.,26.5));
#40039=CARTESIAN_POINT('',(10.,-2.,26.5));
#40040=CARTESIAN_POINT('',(12.5,-2.,26.5));
#40041=CARTESIAN_POINT('Origin',(10.,0.,26.5));
#40042=CARTESIAN_POINT('Origin',(10.,3.397,26.5));
#40043=CARTESIAN_POINT('',(10.,-3.397,26.5));
#40044=CARTESIAN_POINT('Origin',(10.,0.,26.5));
#40045=CARTESIAN_POINT('Origin',(10.05,0.,26.5));
#40046=CARTESIAN_POINT('',(10.1,-3.497,26.5));
#40047=CARTESIAN_POINT('Origin',(10.1,0.,26.5));
#40048=CARTESIAN_POINT('',(10.05,-3.447,26.5));
#40049=CARTESIAN_POINT('Origin',(24.05,0.,26.5));
#40050=CARTESIAN_POINT('',(24.05,-3.497,26.5));
#40051=CARTESIAN_POINT('Origin',(38.96,0.,26.5));
#40052=CARTESIAN_POINT('',(38.92,-1.5612724,26.5));
#40053=CARTESIAN_POINT('',(38.96,-1.6023112,26.5));
#40054=CARTESIAN_POINT('Origin',(38.92,0.,26.5));
#40055=CARTESIAN_POINT('Origin',(33.06,0.,26.5));
#40056=CARTESIAN_POINT('',(27.2,-1.256904,26.5));
#40057=CARTESIAN_POINT('',(33.06,-1.4090882,26.5));
#40058=CARTESIAN_POINT('Origin',(27.2,0.,26.5));
#40059=CARTESIAN_POINT('Origin',(27.2,1.1,26.5));
#40060=CARTESIAN_POINT('',(27.2,-1.1,26.5));
#40061=CARTESIAN_POINT('Origin',(27.2,0.,26.5));
#40062=CARTESIAN_POINT('Origin',(21.1,0.,26.5));
#40063=CARTESIAN_POINT('',(15.,-1.1,26.5));
#40064=CARTESIAN_POINT('',(21.1,-1.1,26.5));
#40065=CARTESIAN_POINT('Origin',(15.,0.,26.5));
#40066=CARTESIAN_POINT('Origin',(15.,2.,26.5));
#76620=UNCERTAINTY_MEASURE_WITH_UNIT(LENGTH_MEASURE(0.001),#76661,
'DISTANCE_ACCURACY_VALUE',
'Maximum model space distance between geometric entities at asserted c
onnectivities');
#76638=UNCERTAINTY_MEASURE_WITH_UNIT(LENGTH_MEASURE(0.001),#76661,
'DISTANCE_ACCURACY_VALUE',
'Maximum model space distance between geometric entities at asserted c
onnectivities');
#76642=(
GEOMETRIC_REPRESENTATION_CONTEXT(3)
GLOBAL_UNCERTAINTY_ASSIGNED_CONTEXT((#76620))
GLOBAL_UNIT_ASSIGNED_CONTEXT((#76661,#76663,#76664))
REPRESENTATION_CONTEXT('','3D')
);
#76660=(
GEOMETRIC_REPRESENTATION_CONTEXT(3)
GLOBAL_UNCERTAINTY_ASSIGNED_CONTEXT((#76638))
GLOBAL_UNIT_ASSIGNED_CONTEXT((#76661,#76663,#76664))
REPRESENTATION_CONTEXT('','3D')
);
#76661=(
LENGTH_UNIT()
NAMED_UNIT(*)
SI_UNIT(.CENTI.,.METRE.)
);
#76663=(
NAMED_UNIT(*)
PLANE_ANGLE_UNIT()
SI_UNIT($,.RADIAN.)
);
#76664=(
NAMED_UNIT(*)
SI_UNIT($,.STERADIAN.)
SOLID_ANGLE_UNIT()
);
#76668=SHAPE_DEFINITION_REPRESENTATION(#76689,#76738);
#76689=PRODUCT_DEFINITION_SHAPE('',$,#76760);
#76738=SHAPE_REPRESENTATION('',(#27395),#76642);
#76756=PRODUCT_DEFINITION_CONTEXT('part definition',#76821,'design');
#76760=PRODUCT_DEFINITION('2026-10-26-11-12-37-453',
'03_Quill_Sleeve_D70_MT4_Socket',#76781,#76756);
#76781=PRODUCT_DEFINITION_FORMATION('',$,#76826);
#76821=APPLICATION_CONTEXT(
'Core Data for Automotive Mechanical Design Process');
#76822=PRODUCT_CONTEXT('part definition',#76821,'mechanical');
#76826=PRODUCT('2026-10-26-11-12-37-453',
'03_Quill_Sleeve_D70_MT4_Socket',$,(#76822));
#76914=COLOUR_RGB('Off White',0.89,0.88,0.83);
#76915=FILL_AREA_STYLE_COLOUR('',#76914);
#76916=FILL_AREA_STYLE('',(#76915));
#76917=SURFACE_STYLE_FILL_AREA(#76916);
#76918=SURFACE_SIDE_STYLE('',(#76917));
#76919=SURFACE_STYLE_USAGE(.BOTH.,#76918);
#76920=PRESENTATION_STYLE_ASSIGNMENT((#76919));
ENDSEC;
END-ISO-10303-21;
